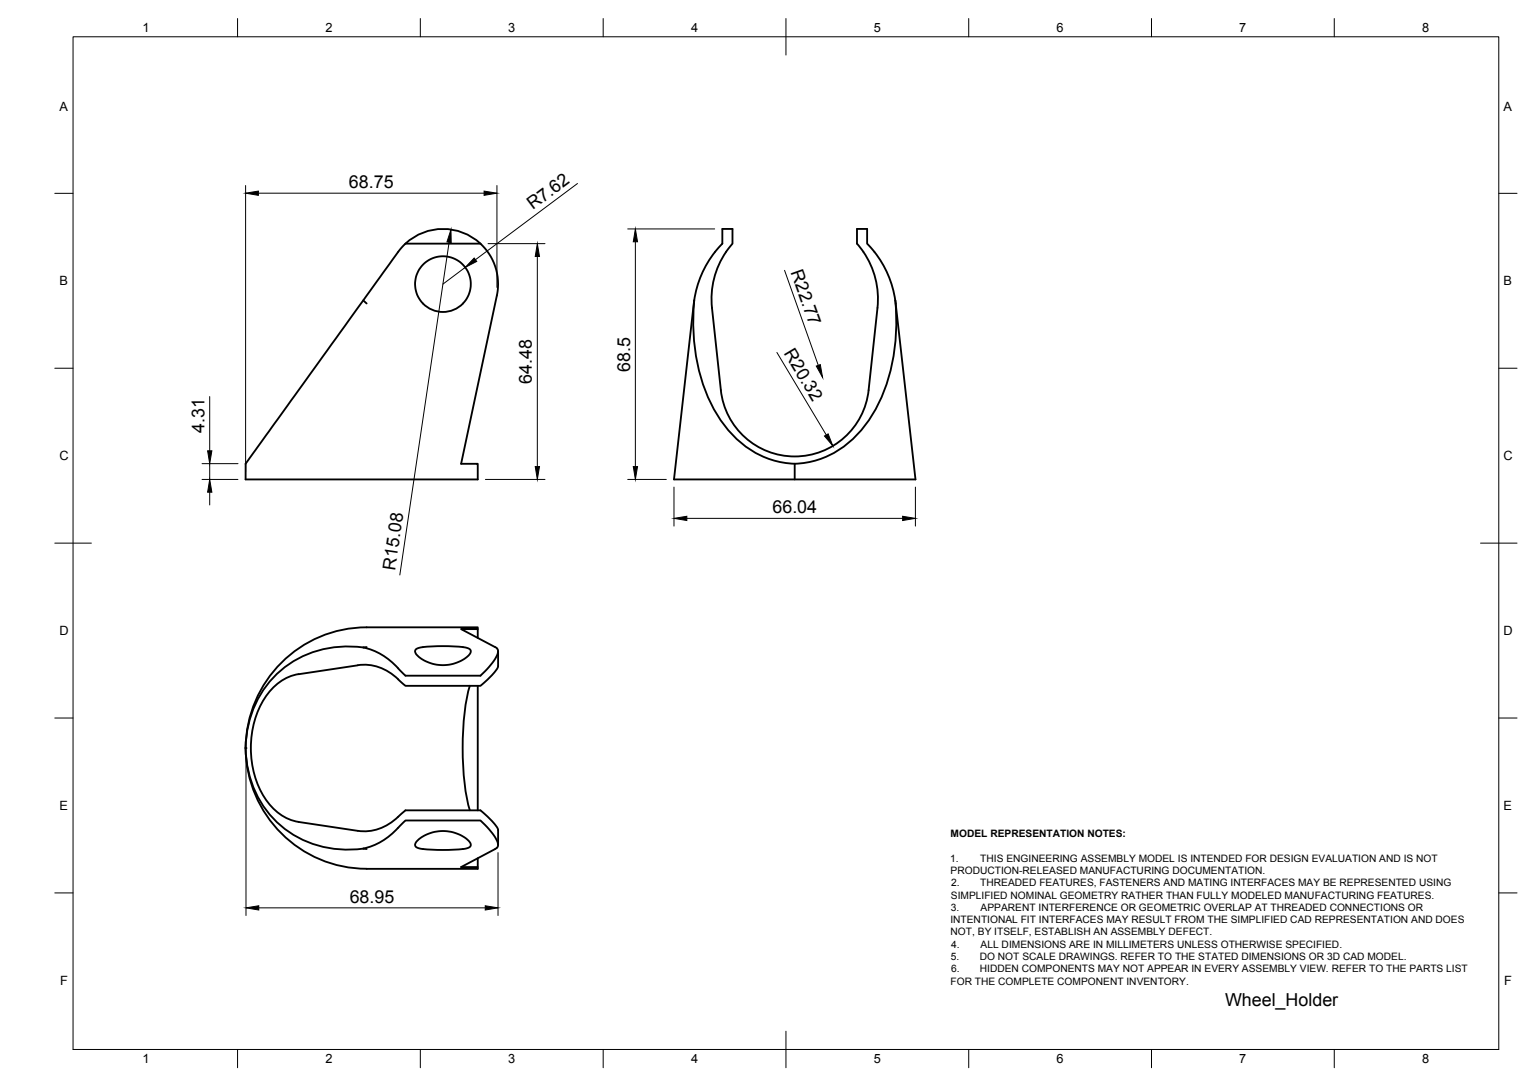
ISO-10303-21;
HEADER;
/* Generated by software containing ST-Developer
 * from STEP Tools, Inc. (www.steptools.com) 
 */

FILE_DESCRIPTION(
/* description */ ('Wheel Holder-Mirrored'),
/* implementation_level */ '2;1');

FILE_NAME(
/* name */ 'Wheel_Holder.step',
/* time_stamp */ '2026-10-07T09:01:46-07:00',
/* author */ (''),
/* organization */ (''),
/* preprocessor_version */ 'ST-DEVELOPER v20.2',
/* originating_system */ 'Autodesk Translation Framework v15.15.0.0',
/* authorisation */ '');

FILE_SCHEMA (('AUTOMOTIVE_DESIGN { 1 0 10303 214 3 1 1 }'));
ENDSEC;

DATA;
#10=MECHANICAL_DESIGN_GEOMETRIC_PRESENTATION_REPRESENTATION('',(#203),#3832);
#59=ELLIPSE('',#1988,0.00766814592499653,0.00762);
#60=ELLIPSE('',#1989,0.0076644002839305,0.00762);
#61=ELLIPSE('',#1993,0.0342294027026876,0.0277785949688766);
#62=ELLIPSE('',#1994,0.028399185304996,0.0277785949688766);
#63=ELLIPSE('',#2002,0.0232756976080203,0.0227670677706907);
#64=ELLIPSE('',#2003,0.0280540873991463,0.0227670677706907);
#65=ELLIPSE('',#2005,0.0232756976080203,0.0227670677706907);
#66=ELLIPSE('',#2006,0.0280540873991463,0.0227670677706907);
#67=ELLIPSE('',#2009,0.0207739608876574,0.02032);
#68=ELLIPSE('',#2010,0.0250387560529214,0.02032);
#69=ELLIPSE('',#2012,0.0076644002839305,0.00762);
#70=ELLIPSE('',#2016,0.0283991853049961,0.0277785949688767);
#71=ELLIPSE('',#2021,0.0570304735096183,0.0331133532215094);
#72=ELLIPSE('',#2022,0.0342294027026876,0.0277785949688767);
#73=ELLIPSE('',#2023,0.0570304735096183,0.0331133532215094);
#74=ELLIPSE('',#2025,0.0333225754026887,0.0331133532215094);
#75=ELLIPSE('',#2026,0.0333225754026887,0.0331133532215094);
#76=ELLIPSE('',#2028,0.00766814592499653,0.00762);
#77=ELLIPSE('',#2034,0.295962272640151,0.0331133532215094);
#170=B_SPLINE_CURVE_WITH_KNOTS('',3,(#3468,#3469,#3470,#3471,#3472,#3473,
#3474,#3475,#3476,#3477,#3478,#3479,#3480,#3481),.UNSPECIFIED.,.F.,.F.,
(4,2,2,2,2,2,4),(0.58453144748271,0.867768183831352,1.16094035782968,1.4691070433662,
1.77727372890272,2.07579244535874,2.37431116181475),.UNSPECIFIED.);
#171=B_SPLINE_CURVE_WITH_KNOTS('',3,(#3484,#3485,#3486,#3487,#3488,#3489,
#3490,#3491,#3492,#3493,#3494,#3495,#3496,#3497),.UNSPECIFIED.,.F.,.F.,
(4,2,2,2,2,2,4),(2.37431116181475,2.66483368462927,2.95535620744379,3.27144000918075,
3.58752381091772,3.88103472550587,4.16394043172282),.UNSPECIFIED.);
#172=B_SPLINE_CURVE_WITH_KNOTS('',3,(#3501,#3502,#3503,#3504,#3505,#3506,
#3507,#3508,#3509,#3510,#3511,#3512,#3513,#3514,#3515,#3516),
 .UNSPECIFIED.,.F.,.F.,(4,2,2,2,2,2,2,4),(-4.27790233879451,-4.09945168810992,
-3.81195458017329,-3.52445747223665,-3.22219845470822,-2.91993943717978,
-2.62905677671056,-2.33817411624134),.UNSPECIFIED.);
#173=B_SPLINE_CURVE_WITH_KNOTS('',3,(#3519,#3520,#3521,#3522,#3523,#3524,
#3525,#3526,#3527,#3528,#3529,#3530,#3531,#3532,#3533,#3534),
 .UNSPECIFIED.,.F.,.F.,(4,2,2,2,2,2,2,4),(-2.33817411624134,-2.04729145577211,
-1.75640879530289,-1.45414977777445,-1.15189076024602,-0.864393652309382,
-0.576896544372747,-0.398445893688138),.UNSPECIFIED.);
#174=B_SPLINE_CURVE_WITH_KNOTS('',3,(#3544,#3545,#3546,#3547,#3548,#3549,
#3550),.UNSPECIFIED.,.F.,.F.,(4,3,4),(-3.65201569549685,-3.58349548702897,
-3.30021421468191),.UNSPECIFIED.);
#175=B_SPLINE_CURVE_WITH_KNOTS('',3,(#3552,#3553,#3554,#3555,#3556,#3557,
#3558,#3559,#3560,#3561,#3562,#3563,#3564,#3565),.UNSPECIFIED.,.F.,.F.,
(4,2,2,2,2,2,4),(-7.77993041753592,-7.7480845912713,-7.46235224345222,-7.12519900195174,
-6.78804576045127,-6.11373927745031,-6.10347024465041),.UNSPECIFIED.);
#176=B_SPLINE_CURVE_WITH_KNOTS('',3,(#3596,#3597,#3598,#3599,#3600,#3601,
#3602,#3603,#3604,#3605,#3606,#3607,#3608,#3609),.UNSPECIFIED.,.F.,.F.,
(4,2,2,2,2,2,4),(-7.66118685225602,-7.63498959168202,-7.35041272704815,
-7.0310473742494,-6.71168202145065,-6.07295131585314,-6.03832591549393),
 .UNSPECIFIED.);
#177=B_SPLINE_CURVE_WITH_KNOTS('',3,(#3611,#3612,#3613,#3614,#3615,#3616),
 .UNSPECIFIED.,.F.,.F.,(4,2,4),(-3.62027438097633,-3.58564898061712,-3.28085403484185),
 .UNSPECIFIED.);
#178=B_SPLINE_CURVE_WITH_KNOTS('',3,(#3628,#3629,#3630,#3631,#3632,#3633,
#3634,#3635,#3636,#3637,#3638,#3639,#3640,#3641,#3642,#3643),
 .UNSPECIFIED.,.F.,.F.,(4,2,2,2,2,2,2,4),(0.398445893688145,0.576896544372747,
0.864393652309382,1.15189076024602,1.45414977777445,1.75640879530289,2.04729145577211,
2.33817411624133),.UNSPECIFIED.);
#179=B_SPLINE_CURVE_WITH_KNOTS('',3,(#3645,#3646,#3647,#3648,#3649,#3650,
#3651,#3652,#3653,#3654,#3655,#3656,#3657,#3658,#3659,#3660),
 .UNSPECIFIED.,.F.,.F.,(4,2,2,2,2,2,2,4),(2.33817411624133,2.62905677671056,
2.91993943717978,3.22219845470822,3.52445747223665,3.81195458017329,4.09945168810992,
4.27790233879452),.UNSPECIFIED.);
#180=B_SPLINE_CURVE_WITH_KNOTS('',3,(#3665,#3666,#3667,#3668,#3669,#3670),
 .UNSPECIFIED.,.F.,.F.,(4,2,4),(-6.38055499661601,-6.10670626645482,-6.04021537866389),
 .UNSPECIFIED.);
#181=B_SPLINE_CURVE_WITH_KNOTS('',3,(#3671,#3672,#3673,#3674,#3675,#3676,
#3677,#3678,#3679,#3680,#3681,#3682,#3683,#3684),.UNSPECIFIED.,.F.,.F.,
(4,2,2,2,2,2,4),(-3.62027438097633,-3.58564898061712,-2.94691827501961,
-2.62755292222086,-2.30818756942211,-2.02361070478824,-1.99741344421424),
 .UNSPECIFIED.);
#182=B_SPLINE_CURVE_WITH_KNOTS('',3,(#3724,#3725,#3726,#3727,#3728,#3729,
#3730),.UNSPECIFIED.,.F.,.F.,(4,3,4),(3.30021421468192,3.58349548702897,
3.65201569549685),.UNSPECIFIED.);
#183=B_SPLINE_CURVE_WITH_KNOTS('',3,(#3733,#3734,#3735,#3736,#3737,#3738,
#3739,#3740,#3741,#3742,#3743,#3744,#3745,#3746),.UNSPECIFIED.,.F.,.F.,
(4,2,2,2,2,2,4),(6.10060038618841,6.11086941898832,6.78517590198927,7.12232914348975,
7.45948238499022,7.7452147328093,7.77706055907392),.UNSPECIFIED.);
#184=B_SPLINE_CURVE_WITH_KNOTS('',3,(#3763,#3764,#3765,#3766,#3767,#3768,
#3769,#3770,#3771,#3772,#3773,#3774,#3775,#3776),.UNSPECIFIED.,.F.,.F.,
(4,2,2,2,2,2,4),(0.584524822753337,0.867430528970284,1.16094144355843,1.4770252452954,
1.79310904703237,2.08363156984688,2.3741540926614),.UNSPECIFIED.);
#185=B_SPLINE_CURVE_WITH_KNOTS('',3,(#3779,#3780,#3781,#3782,#3783,#3784,
#3785,#3786,#3787,#3788,#3789,#3790,#3791,#3792),.UNSPECIFIED.,.F.,.F.,
(4,2,2,2,2,2,4),(2.3741540926614,2.66467661547592,2.95519913829043,3.2712829400274,
3.58736674176437,3.88087765635252,4.16378336256947),.UNSPECIFIED.);
#191=SHAPE_REPRESENTATION_RELATIONSHIP('SRR','None',#3868,#197);
#197=ADVANCED_BREP_SHAPE_REPRESENTATION('',(#209),#3831);
#203=STYLED_ITEM('',(#3906),#209);
#209=MANIFOLD_SOLID_BREP('Body1',#1788);
#260=PLANE('',#1990);
#261=PLANE('',#1996);
#262=PLANE('',#1997);
#263=PLANE('',#1999);
#264=PLANE('',#2007);
#265=PLANE('',#2011);
#266=PLANE('',#2013);
#267=PLANE('',#2014);
#268=PLANE('',#2015);
#269=PLANE('',#2020);
#270=PLANE('',#2024);
#271=PLANE('',#2029);
#272=PLANE('',#2032);
#353=FACE_OUTER_BOUND('',#474,.T.);
#354=FACE_OUTER_BOUND('',#475,.T.);
#355=FACE_OUTER_BOUND('',#476,.T.);
#356=FACE_OUTER_BOUND('',#477,.T.);
#357=FACE_OUTER_BOUND('',#478,.T.);
#358=FACE_OUTER_BOUND('',#479,.T.);
#359=FACE_OUTER_BOUND('',#480,.T.);
#360=FACE_OUTER_BOUND('',#481,.T.);
#361=FACE_OUTER_BOUND('',#482,.T.);
#362=FACE_OUTER_BOUND('',#483,.T.);
#363=FACE_OUTER_BOUND('',#484,.T.);
#364=FACE_OUTER_BOUND('',#485,.T.);
#365=FACE_OUTER_BOUND('',#486,.T.);
#366=FACE_OUTER_BOUND('',#487,.T.);
#367=FACE_OUTER_BOUND('',#488,.T.);
#368=FACE_OUTER_BOUND('',#489,.T.);
#369=FACE_OUTER_BOUND('',#490,.T.);
#370=FACE_OUTER_BOUND('',#491,.T.);
#371=FACE_OUTER_BOUND('',#492,.T.);
#372=FACE_OUTER_BOUND('',#493,.T.);
#373=FACE_OUTER_BOUND('',#494,.T.);
#374=FACE_OUTER_BOUND('',#495,.T.);
#375=FACE_OUTER_BOUND('',#496,.T.);
#376=FACE_OUTER_BOUND('',#497,.T.);
#474=EDGE_LOOP('',(#1497,#1498,#1499,#1500,#1501,#1502,#1503,#1504));
#475=EDGE_LOOP('',(#1505,#1506));
#476=EDGE_LOOP('',(#1507,#1508,#1509,#1510,#1511,#1512,#1513,#1514,#1515,
#1516));
#477=EDGE_LOOP('',(#1517,#1518,#1519,#1520,#1521,#1522,#1523,#1524));
#478=EDGE_LOOP('',(#1525,#1526));
#479=EDGE_LOOP('',(#1527,#1528));
#480=EDGE_LOOP('',(#1529,#1530,#1531,#1532,#1533,#1534,#1535,#1536,#1537));
#481=EDGE_LOOP('',(#1538,#1539,#1540,#1541,#1542,#1543,#1544,#1545,#1546));
#482=EDGE_LOOP('',(#1547,#1548,#1549,#1550,#1551,#1552));
#483=EDGE_LOOP('',(#1553,#1554,#1555,#1556));
#484=EDGE_LOOP('',(#1557,#1558,#1559,#1560,#1561,#1562));
#485=EDGE_LOOP('',(#1563,#1564,#1565,#1566));
#486=EDGE_LOOP('',(#1567,#1568,#1569,#1570));
#487=EDGE_LOOP('',(#1571,#1572,#1573,#1574,#1575,#1576,#1577,#1578,#1579,
#1580,#1581,#1582));
#488=EDGE_LOOP('',(#1583,#1584,#1585,#1586,#1587,#1588,#1589,#1590));
#489=EDGE_LOOP('',(#1591,#1592,#1593,#1594,#1595,#1596,#1597,#1598));
#490=EDGE_LOOP('',(#1599,#1600,#1601,#1602,#1603,#1604,#1605,#1606,#1607,
#1608,#1609));
#491=EDGE_LOOP('',(#1610,#1611,#1612,#1613,#1614));
#492=EDGE_LOOP('',(#1615,#1616,#1617,#1618,#1619,#1620,#1621,#1622));
#493=EDGE_LOOP('',(#1623,#1624));
#494=EDGE_LOOP('',(#1625,#1626,#1627,#1628,#1629,#1630,#1631,#1632,#1633,
#1634));
#495=EDGE_LOOP('',(#1635,#1636,#1637,#1638,#1639,#1640,#1641,#1642));
#496=EDGE_LOOP('',(#1643,#1644,#1645,#1646,#1647));
#497=EDGE_LOOP('',(#1648,#1649,#1650,#1651,#1652));
#554=LINE('',#3499,#647);
#555=LINE('',#3538,#648);
#556=LINE('',#3568,#649);
#557=LINE('',#3570,#650);
#558=LINE('',#3574,#651);
#559=LINE('',#3576,#652);
#560=LINE('',#3578,#653);
#561=LINE('',#3580,#654);
#562=LINE('',#3581,#655);
#563=LINE('',#3585,#656);
#564=LINE('',#3591,#657);
#565=LINE('',#3619,#658);
#566=LINE('',#3620,#659);
#567=LINE('',#3626,#660);
#568=LINE('',#3662,#661);
#569=LINE('',#3688,#662);
#570=LINE('',#3689,#663);
#571=LINE('',#3690,#664);
#572=LINE('',#3696,#665);
#573=LINE('',#3698,#666);
#574=LINE('',#3699,#667);
#575=LINE('',#3703,#668);
#576=LINE('',#3705,#669);
#577=LINE('',#3706,#670);
#578=LINE('',#3709,#671);
#579=LINE('',#3710,#672);
#580=LINE('',#3713,#673);
#581=LINE('',#3716,#674);
#582=LINE('',#3717,#675);
#583=LINE('',#3719,#676);
#584=LINE('',#3722,#677);
#585=LINE('',#3755,#678);
#586=LINE('',#3761,#679);
#587=LINE('',#3794,#680);
#588=LINE('',#3797,#681);
#589=LINE('',#3798,#682);
#590=LINE('',#3801,#683);
#647=VECTOR('',#2370,0.00762);
#648=VECTOR('',#2375,1.);
#649=VECTOR('',#2384,1.);
#650=VECTOR('',#2385,1.);
#651=VECTOR('',#2390,1.);
#652=VECTOR('',#2391,1.);
#653=VECTOR('',#2392,1.);
#654=VECTOR('',#2393,1.);
#655=VECTOR('',#2394,1.);
#656=VECTOR('',#2397,1.);
#657=VECTOR('',#2404,1.);
#658=VECTOR('',#2411,1.);
#659=VECTOR('',#2412,1.);
#660=VECTOR('',#2417,1.);
#661=VECTOR('',#2418,1.);
#662=VECTOR('',#2423,1.);
#663=VECTOR('',#2424,1.);
#664=VECTOR('',#2425,1.);
#665=VECTOR('',#2432,1.);
#666=VECTOR('',#2435,1.);
#667=VECTOR('',#2436,1.);
#668=VECTOR('',#2441,1.);
#669=VECTOR('',#2442,1.);
#670=VECTOR('',#2443,1.);
#671=VECTOR('',#2446,1.);
#672=VECTOR('',#2447,1.);
#673=VECTOR('',#2450,1.);
#674=VECTOR('',#2453,1.);
#675=VECTOR('',#2454,1.);
#676=VECTOR('',#2457,1.);
#677=VECTOR('',#2460,1.);
#678=VECTOR('',#2473,1.);
#679=VECTOR('',#2480,0.00762);
#680=VECTOR('',#2485,1.);
#681=VECTOR('',#2488,1.);
#682=VECTOR('',#2489,1.);
#683=VECTOR('',#2494,1.);
#740=CIRCLE('',#1991,0.01508125);
#741=CIRCLE('',#1995,0.0608802828924915);
#742=CIRCLE('',#1998,0.01508125);
#743=CIRCLE('',#2000,0.01508125);
#744=CIRCLE('',#2019,0.01508125);
#745=CIRCLE('',#2031,0.0608802828794672);
#851=VERTEX_POINT('',#3466);
#852=VERTEX_POINT('',#3467);
#853=VERTEX_POINT('',#3482);
#854=VERTEX_POINT('',#3498);
#855=VERTEX_POINT('',#3500);
#856=VERTEX_POINT('',#3517);
#857=VERTEX_POINT('',#3536);
#858=VERTEX_POINT('',#3537);
#859=VERTEX_POINT('',#3541);
#860=VERTEX_POINT('',#3542);
#861=VERTEX_POINT('',#3551);
#862=VERTEX_POINT('',#3566);
#863=VERTEX_POINT('',#3569);
#864=VERTEX_POINT('',#3573);
#865=VERTEX_POINT('',#3575);
#866=VERTEX_POINT('',#3577);
#867=VERTEX_POINT('',#3579);
#868=VERTEX_POINT('',#3583);
#869=VERTEX_POINT('',#3584);
#870=VERTEX_POINT('',#3588);
#871=VERTEX_POINT('',#3589);
#872=VERTEX_POINT('',#3593);
#873=VERTEX_POINT('',#3594);
#874=VERTEX_POINT('',#3610);
#875=VERTEX_POINT('',#3617);
#876=VERTEX_POINT('',#3622);
#877=VERTEX_POINT('',#3623);
#878=VERTEX_POINT('',#3625);
#879=VERTEX_POINT('',#3627);
#880=VERTEX_POINT('',#3644);
#881=VERTEX_POINT('',#3661);
#882=VERTEX_POINT('',#3663);
#883=VERTEX_POINT('',#3686);
#884=VERTEX_POINT('',#3687);
#885=VERTEX_POINT('',#3692);
#886=VERTEX_POINT('',#3694);
#887=VERTEX_POINT('',#3702);
#888=VERTEX_POINT('',#3704);
#889=VERTEX_POINT('',#3708);
#890=VERTEX_POINT('',#3712);
#891=VERTEX_POINT('',#3714);
#892=VERTEX_POINT('',#3721);
#893=VERTEX_POINT('',#3723);
#894=VERTEX_POINT('',#3731);
#895=VERTEX_POINT('',#3748);
#896=VERTEX_POINT('',#3749);
#897=VERTEX_POINT('',#3754);
#898=VERTEX_POINT('',#3756);
#899=VERTEX_POINT('',#3760);
#900=VERTEX_POINT('',#3762);
#901=VERTEX_POINT('',#3777);
#902=VERTEX_POINT('',#3796);
#1075=EDGE_CURVE('',#851,#852,#170,.T.);
#1076=EDGE_CURVE('',#853,#851,#59,.T.);
#1077=EDGE_CURVE('',#852,#853,#171,.T.);
#1078=EDGE_CURVE('',#852,#854,#554,.T.);
#1079=EDGE_CURVE('',#854,#855,#172,.F.);
#1080=EDGE_CURVE('',#856,#855,#60,.T.);
#1081=EDGE_CURVE('',#856,#854,#173,.F.);
#1082=EDGE_CURVE('',#857,#858,#555,.T.);
#1083=EDGE_CURVE('',#857,#858,#740,.T.);
#1084=EDGE_CURVE('',#859,#860,#61,.T.);
#1085=EDGE_CURVE('',#857,#860,#174,.T.);
#1086=EDGE_CURVE('',#861,#858,#175,.T.);
#1087=EDGE_CURVE('',#861,#862,#62,.T.);
#1088=EDGE_CURVE('',#851,#862,#556,.T.);
#1089=EDGE_CURVE('',#863,#853,#557,.T.);
#1090=EDGE_CURVE('',#859,#863,#741,.T.);
#1091=EDGE_CURVE('',#862,#864,#558,.T.);
#1092=EDGE_CURVE('',#864,#865,#559,.T.);
#1093=EDGE_CURVE('',#865,#866,#560,.T.);
#1094=EDGE_CURVE('',#867,#866,#561,.T.);
#1095=EDGE_CURVE('',#863,#867,#562,.F.);
#1096=EDGE_CURVE('',#868,#869,#563,.T.);
#1097=EDGE_CURVE('',#868,#869,#742,.T.);
#1098=EDGE_CURVE('',#870,#871,#743,.T.);
#1099=EDGE_CURVE('',#871,#870,#564,.T.);
#1100=EDGE_CURVE('',#872,#873,#63,.T.);
#1101=EDGE_CURVE('',#872,#870,#176,.T.);
#1102=EDGE_CURVE('',#871,#874,#177,.T.);
#1103=EDGE_CURVE('',#875,#874,#64,.T.);
#1104=EDGE_CURVE('',#875,#855,#565,.T.);
#1105=EDGE_CURVE('',#856,#873,#566,.T.);
#1106=EDGE_CURVE('',#876,#877,#65,.T.);
#1107=EDGE_CURVE('',#878,#876,#567,.T.);
#1108=EDGE_CURVE('',#879,#878,#178,.F.);
#1109=EDGE_CURVE('',#880,#879,#179,.F.);
#1110=EDGE_CURVE('',#881,#880,#568,.T.);
#1111=EDGE_CURVE('',#882,#881,#66,.T.);
#1112=EDGE_CURVE('',#882,#868,#180,.T.);
#1113=EDGE_CURVE('',#869,#877,#181,.T.);
#1114=EDGE_CURVE('',#883,#884,#569,.T.);
#1115=EDGE_CURVE('',#884,#873,#570,.T.);
#1116=EDGE_CURVE('',#875,#883,#571,.T.);
#1117=EDGE_CURVE('',#884,#885,#67,.T.);
#1118=EDGE_CURVE('',#886,#883,#68,.T.);
#1119=EDGE_CURVE('',#886,#885,#572,.T.);
#1120=EDGE_CURVE('',#885,#876,#573,.T.);
#1121=EDGE_CURVE('',#881,#886,#574,.T.);
#1122=EDGE_CURVE('',#878,#880,#69,.T.);
#1123=EDGE_CURVE('',#865,#887,#575,.T.);
#1124=EDGE_CURVE('',#888,#887,#576,.T.);
#1125=EDGE_CURVE('',#866,#888,#577,.T.);
#1126=EDGE_CURVE('',#864,#889,#578,.T.);
#1127=EDGE_CURVE('',#887,#889,#579,.T.);
#1128=EDGE_CURVE('',#877,#890,#580,.T.);
#1129=EDGE_CURVE('',#891,#890,#70,.T.);
#1130=EDGE_CURVE('',#889,#891,#581,.T.);
#1131=EDGE_CURVE('',#861,#872,#582,.T.);
#1132=EDGE_CURVE('',#860,#874,#583,.T.);
#1133=EDGE_CURVE('',#882,#892,#584,.T.);
#1134=EDGE_CURVE('',#892,#893,#182,.T.);
#1135=EDGE_CURVE('',#894,#893,#744,.T.);
#1136=EDGE_CURVE('',#894,#890,#183,.T.);
#1137=EDGE_CURVE('',#895,#896,#71,.T.);
#1138=EDGE_CURVE('',#892,#895,#72,.T.);
#1139=EDGE_CURVE('',#896,#859,#73,.T.);
#1140=EDGE_CURVE('',#897,#888,#585,.T.);
#1141=EDGE_CURVE('',#898,#897,#74,.F.);
#1142=EDGE_CURVE('',#867,#898,#75,.F.);
#1143=EDGE_CURVE('',#879,#899,#586,.T.);
#1144=EDGE_CURVE('',#900,#899,#184,.T.);
#1145=EDGE_CURVE('',#901,#900,#76,.T.);
#1146=EDGE_CURVE('',#899,#901,#185,.T.);
#1147=EDGE_CURVE('',#893,#894,#587,.T.);
#1148=EDGE_CURVE('',#902,#900,#588,.T.);
#1149=EDGE_CURVE('',#901,#891,#589,.T.);
#1150=EDGE_CURVE('',#902,#895,#745,.F.);
#1151=EDGE_CURVE('',#897,#902,#590,.F.);
#1152=EDGE_CURVE('',#896,#898,#77,.F.);
#1497=ORIENTED_EDGE('',*,*,#1075,.F.);
#1498=ORIENTED_EDGE('',*,*,#1076,.F.);
#1499=ORIENTED_EDGE('',*,*,#1077,.F.);
#1500=ORIENTED_EDGE('',*,*,#1078,.T.);
#1501=ORIENTED_EDGE('',*,*,#1079,.T.);
#1502=ORIENTED_EDGE('',*,*,#1080,.F.);
#1503=ORIENTED_EDGE('',*,*,#1081,.T.);
#1504=ORIENTED_EDGE('',*,*,#1078,.F.);
#1505=ORIENTED_EDGE('',*,*,#1082,.F.);
#1506=ORIENTED_EDGE('',*,*,#1083,.T.);
#1507=ORIENTED_EDGE('',*,*,#1084,.T.);
#1508=ORIENTED_EDGE('',*,*,#1085,.F.);
#1509=ORIENTED_EDGE('',*,*,#1082,.T.);
#1510=ORIENTED_EDGE('',*,*,#1086,.F.);
#1511=ORIENTED_EDGE('',*,*,#1087,.T.);
#1512=ORIENTED_EDGE('',*,*,#1088,.F.);
#1513=ORIENTED_EDGE('',*,*,#1075,.T.);
#1514=ORIENTED_EDGE('',*,*,#1077,.T.);
#1515=ORIENTED_EDGE('',*,*,#1089,.F.);
#1516=ORIENTED_EDGE('',*,*,#1090,.F.);
#1517=ORIENTED_EDGE('',*,*,#1089,.T.);
#1518=ORIENTED_EDGE('',*,*,#1076,.T.);
#1519=ORIENTED_EDGE('',*,*,#1088,.T.);
#1520=ORIENTED_EDGE('',*,*,#1091,.T.);
#1521=ORIENTED_EDGE('',*,*,#1092,.T.);
#1522=ORIENTED_EDGE('',*,*,#1093,.T.);
#1523=ORIENTED_EDGE('',*,*,#1094,.F.);
#1524=ORIENTED_EDGE('',*,*,#1095,.F.);
#1525=ORIENTED_EDGE('',*,*,#1096,.F.);
#1526=ORIENTED_EDGE('',*,*,#1097,.T.);
#1527=ORIENTED_EDGE('',*,*,#1098,.T.);
#1528=ORIENTED_EDGE('',*,*,#1099,.T.);
#1529=ORIENTED_EDGE('',*,*,#1100,.F.);
#1530=ORIENTED_EDGE('',*,*,#1101,.T.);
#1531=ORIENTED_EDGE('',*,*,#1099,.F.);
#1532=ORIENTED_EDGE('',*,*,#1102,.T.);
#1533=ORIENTED_EDGE('',*,*,#1103,.F.);
#1534=ORIENTED_EDGE('',*,*,#1104,.T.);
#1535=ORIENTED_EDGE('',*,*,#1079,.F.);
#1536=ORIENTED_EDGE('',*,*,#1081,.F.);
#1537=ORIENTED_EDGE('',*,*,#1105,.T.);
#1538=ORIENTED_EDGE('',*,*,#1106,.F.);
#1539=ORIENTED_EDGE('',*,*,#1107,.F.);
#1540=ORIENTED_EDGE('',*,*,#1108,.F.);
#1541=ORIENTED_EDGE('',*,*,#1109,.F.);
#1542=ORIENTED_EDGE('',*,*,#1110,.F.);
#1543=ORIENTED_EDGE('',*,*,#1111,.F.);
#1544=ORIENTED_EDGE('',*,*,#1112,.T.);
#1545=ORIENTED_EDGE('',*,*,#1096,.T.);
#1546=ORIENTED_EDGE('',*,*,#1113,.T.);
#1547=ORIENTED_EDGE('',*,*,#1114,.T.);
#1548=ORIENTED_EDGE('',*,*,#1115,.T.);
#1549=ORIENTED_EDGE('',*,*,#1105,.F.);
#1550=ORIENTED_EDGE('',*,*,#1080,.T.);
#1551=ORIENTED_EDGE('',*,*,#1104,.F.);
#1552=ORIENTED_EDGE('',*,*,#1116,.T.);
#1553=ORIENTED_EDGE('',*,*,#1117,.F.);
#1554=ORIENTED_EDGE('',*,*,#1114,.F.);
#1555=ORIENTED_EDGE('',*,*,#1118,.F.);
#1556=ORIENTED_EDGE('',*,*,#1119,.T.);
#1557=ORIENTED_EDGE('',*,*,#1120,.F.);
#1558=ORIENTED_EDGE('',*,*,#1119,.F.);
#1559=ORIENTED_EDGE('',*,*,#1121,.F.);
#1560=ORIENTED_EDGE('',*,*,#1110,.T.);
#1561=ORIENTED_EDGE('',*,*,#1122,.F.);
#1562=ORIENTED_EDGE('',*,*,#1107,.T.);
#1563=ORIENTED_EDGE('',*,*,#1123,.T.);
#1564=ORIENTED_EDGE('',*,*,#1124,.F.);
#1565=ORIENTED_EDGE('',*,*,#1125,.F.);
#1566=ORIENTED_EDGE('',*,*,#1093,.F.);
#1567=ORIENTED_EDGE('',*,*,#1126,.T.);
#1568=ORIENTED_EDGE('',*,*,#1127,.F.);
#1569=ORIENTED_EDGE('',*,*,#1123,.F.);
#1570=ORIENTED_EDGE('',*,*,#1092,.F.);
#1571=ORIENTED_EDGE('',*,*,#1100,.T.);
#1572=ORIENTED_EDGE('',*,*,#1115,.F.);
#1573=ORIENTED_EDGE('',*,*,#1117,.T.);
#1574=ORIENTED_EDGE('',*,*,#1120,.T.);
#1575=ORIENTED_EDGE('',*,*,#1106,.T.);
#1576=ORIENTED_EDGE('',*,*,#1128,.T.);
#1577=ORIENTED_EDGE('',*,*,#1129,.F.);
#1578=ORIENTED_EDGE('',*,*,#1130,.F.);
#1579=ORIENTED_EDGE('',*,*,#1126,.F.);
#1580=ORIENTED_EDGE('',*,*,#1091,.F.);
#1581=ORIENTED_EDGE('',*,*,#1087,.F.);
#1582=ORIENTED_EDGE('',*,*,#1131,.T.);
#1583=ORIENTED_EDGE('',*,*,#1101,.F.);
#1584=ORIENTED_EDGE('',*,*,#1131,.F.);
#1585=ORIENTED_EDGE('',*,*,#1086,.T.);
#1586=ORIENTED_EDGE('',*,*,#1083,.F.);
#1587=ORIENTED_EDGE('',*,*,#1085,.T.);
#1588=ORIENTED_EDGE('',*,*,#1132,.T.);
#1589=ORIENTED_EDGE('',*,*,#1102,.F.);
#1590=ORIENTED_EDGE('',*,*,#1098,.F.);
#1591=ORIENTED_EDGE('',*,*,#1133,.T.);
#1592=ORIENTED_EDGE('',*,*,#1134,.T.);
#1593=ORIENTED_EDGE('',*,*,#1135,.F.);
#1594=ORIENTED_EDGE('',*,*,#1136,.T.);
#1595=ORIENTED_EDGE('',*,*,#1128,.F.);
#1596=ORIENTED_EDGE('',*,*,#1113,.F.);
#1597=ORIENTED_EDGE('',*,*,#1097,.F.);
#1598=ORIENTED_EDGE('',*,*,#1112,.F.);
#1599=ORIENTED_EDGE('',*,*,#1137,.F.);
#1600=ORIENTED_EDGE('',*,*,#1138,.F.);
#1601=ORIENTED_EDGE('',*,*,#1133,.F.);
#1602=ORIENTED_EDGE('',*,*,#1111,.T.);
#1603=ORIENTED_EDGE('',*,*,#1121,.T.);
#1604=ORIENTED_EDGE('',*,*,#1118,.T.);
#1605=ORIENTED_EDGE('',*,*,#1116,.F.);
#1606=ORIENTED_EDGE('',*,*,#1103,.T.);
#1607=ORIENTED_EDGE('',*,*,#1132,.F.);
#1608=ORIENTED_EDGE('',*,*,#1084,.F.);
#1609=ORIENTED_EDGE('',*,*,#1139,.F.);
#1610=ORIENTED_EDGE('',*,*,#1094,.T.);
#1611=ORIENTED_EDGE('',*,*,#1125,.T.);
#1612=ORIENTED_EDGE('',*,*,#1140,.F.);
#1613=ORIENTED_EDGE('',*,*,#1141,.F.);
#1614=ORIENTED_EDGE('',*,*,#1142,.F.);
#1615=ORIENTED_EDGE('',*,*,#1109,.T.);
#1616=ORIENTED_EDGE('',*,*,#1143,.T.);
#1617=ORIENTED_EDGE('',*,*,#1144,.F.);
#1618=ORIENTED_EDGE('',*,*,#1145,.F.);
#1619=ORIENTED_EDGE('',*,*,#1146,.F.);
#1620=ORIENTED_EDGE('',*,*,#1143,.F.);
#1621=ORIENTED_EDGE('',*,*,#1108,.T.);
#1622=ORIENTED_EDGE('',*,*,#1122,.T.);
#1623=ORIENTED_EDGE('',*,*,#1135,.T.);
#1624=ORIENTED_EDGE('',*,*,#1147,.T.);
#1625=ORIENTED_EDGE('',*,*,#1148,.T.);
#1626=ORIENTED_EDGE('',*,*,#1144,.T.);
#1627=ORIENTED_EDGE('',*,*,#1146,.T.);
#1628=ORIENTED_EDGE('',*,*,#1149,.T.);
#1629=ORIENTED_EDGE('',*,*,#1129,.T.);
#1630=ORIENTED_EDGE('',*,*,#1136,.F.);
#1631=ORIENTED_EDGE('',*,*,#1147,.F.);
#1632=ORIENTED_EDGE('',*,*,#1134,.F.);
#1633=ORIENTED_EDGE('',*,*,#1138,.T.);
#1634=ORIENTED_EDGE('',*,*,#1150,.F.);
#1635=ORIENTED_EDGE('',*,*,#1140,.T.);
#1636=ORIENTED_EDGE('',*,*,#1124,.T.);
#1637=ORIENTED_EDGE('',*,*,#1127,.T.);
#1638=ORIENTED_EDGE('',*,*,#1130,.T.);
#1639=ORIENTED_EDGE('',*,*,#1149,.F.);
#1640=ORIENTED_EDGE('',*,*,#1145,.T.);
#1641=ORIENTED_EDGE('',*,*,#1148,.F.);
#1642=ORIENTED_EDGE('',*,*,#1151,.F.);
#1643=ORIENTED_EDGE('',*,*,#1151,.T.);
#1644=ORIENTED_EDGE('',*,*,#1150,.T.);
#1645=ORIENTED_EDGE('',*,*,#1137,.T.);
#1646=ORIENTED_EDGE('',*,*,#1152,.T.);
#1647=ORIENTED_EDGE('',*,*,#1141,.T.);
#1648=ORIENTED_EDGE('',*,*,#1142,.T.);
#1649=ORIENTED_EDGE('',*,*,#1152,.F.);
#1650=ORIENTED_EDGE('',*,*,#1139,.T.);
#1651=ORIENTED_EDGE('',*,*,#1090,.T.);
#1652=ORIENTED_EDGE('',*,*,#1095,.T.);
#1668=CYLINDRICAL_SURFACE('',#1987,0.00762);
#1669=CYLINDRICAL_SURFACE('',#1992,0.0277785949688766);
#1670=CYLINDRICAL_SURFACE('',#2001,0.0227670677706907);
#1671=CYLINDRICAL_SURFACE('',#2004,0.0227670677706907);
#1672=CYLINDRICAL_SURFACE('',#2008,0.02032);
#1673=CYLINDRICAL_SURFACE('',#2017,0.01508125);
#1674=CYLINDRICAL_SURFACE('',#2018,0.01508125);
#1675=CYLINDRICAL_SURFACE('',#2027,0.00762);
#1676=CYLINDRICAL_SURFACE('',#2030,0.0277785949688767);
#1677=CYLINDRICAL_SURFACE('',#2033,0.0331133532215094);
#1678=CYLINDRICAL_SURFACE('',#2035,0.0331133532215094);
#1759=ADVANCED_FACE('',(#353),#1668,.F.);
#1760=ADVANCED_FACE('',(#354),#260,.F.);
#1761=ADVANCED_FACE('',(#355),#1669,.T.);
#1762=ADVANCED_FACE('',(#356),#261,.T.);
#1763=ADVANCED_FACE('',(#357),#262,.F.);
#1764=ADVANCED_FACE('',(#358),#263,.F.);
#1765=ADVANCED_FACE('',(#359),#1670,.F.);
#1766=ADVANCED_FACE('',(#360),#1671,.F.);
#1767=ADVANCED_FACE('',(#361),#264,.T.);
#1768=ADVANCED_FACE('',(#362),#1672,.F.);
#1769=ADVANCED_FACE('',(#363),#265,.F.);
#1770=ADVANCED_FACE('',(#364),#266,.T.);
#1771=ADVANCED_FACE('',(#365),#267,.T.);
#1772=ADVANCED_FACE('',(#366),#268,.T.);
#1773=ADVANCED_FACE('',(#367),#1673,.T.);
#1774=ADVANCED_FACE('',(#368),#1674,.T.);
#1775=ADVANCED_FACE('',(#369),#269,.T.);
#1776=ADVANCED_FACE('',(#370),#270,.F.);
#1777=ADVANCED_FACE('',(#371),#1675,.F.);
#1778=ADVANCED_FACE('',(#372),#271,.F.);
#1779=ADVANCED_FACE('',(#373),#1676,.T.);
#1780=ADVANCED_FACE('',(#374),#272,.T.);
#1781=ADVANCED_FACE('',(#375),#1677,.T.);
#1782=ADVANCED_FACE('',(#376),#1678,.T.);
#1788=CLOSED_SHELL('',(#1759,#1760,#1761,#1762,#1763,#1764,#1765,#1766,
#1767,#1768,#1769,#1770,#1771,#1772,#1773,#1774,#1775,#1776,#1777,#1778,
#1779,#1780,#1781,#1782));
#1986=AXIS2_PLACEMENT_3D('',#3464,#2364,#2365);
#1987=AXIS2_PLACEMENT_3D('',#3465,#2366,#2367);
#1988=AXIS2_PLACEMENT_3D('',#3483,#2368,#2369);
#1989=AXIS2_PLACEMENT_3D('',#3518,#2371,#2372);
#1990=AXIS2_PLACEMENT_3D('',#3535,#2373,#2374);
#1991=AXIS2_PLACEMENT_3D('',#3539,#2376,#2377);
#1992=AXIS2_PLACEMENT_3D('',#3540,#2378,#2379);
#1993=AXIS2_PLACEMENT_3D('',#3543,#2380,#2381);
#1994=AXIS2_PLACEMENT_3D('',#3567,#2382,#2383);
#1995=AXIS2_PLACEMENT_3D('',#3571,#2386,#2387);
#1996=AXIS2_PLACEMENT_3D('',#3572,#2388,#2389);
#1997=AXIS2_PLACEMENT_3D('',#3582,#2395,#2396);
#1998=AXIS2_PLACEMENT_3D('',#3586,#2398,#2399);
#1999=AXIS2_PLACEMENT_3D('',#3587,#2400,#2401);
#2000=AXIS2_PLACEMENT_3D('',#3590,#2402,#2403);
#2001=AXIS2_PLACEMENT_3D('',#3592,#2405,#2406);
#2002=AXIS2_PLACEMENT_3D('',#3595,#2407,#2408);
#2003=AXIS2_PLACEMENT_3D('',#3618,#2409,#2410);
#2004=AXIS2_PLACEMENT_3D('',#3621,#2413,#2414);
#2005=AXIS2_PLACEMENT_3D('',#3624,#2415,#2416);
#2006=AXIS2_PLACEMENT_3D('',#3664,#2419,#2420);
#2007=AXIS2_PLACEMENT_3D('',#3685,#2421,#2422);
#2008=AXIS2_PLACEMENT_3D('',#3691,#2426,#2427);
#2009=AXIS2_PLACEMENT_3D('',#3693,#2428,#2429);
#2010=AXIS2_PLACEMENT_3D('',#3695,#2430,#2431);
#2011=AXIS2_PLACEMENT_3D('',#3697,#2433,#2434);
#2012=AXIS2_PLACEMENT_3D('',#3700,#2437,#2438);
#2013=AXIS2_PLACEMENT_3D('',#3701,#2439,#2440);
#2014=AXIS2_PLACEMENT_3D('',#3707,#2444,#2445);
#2015=AXIS2_PLACEMENT_3D('',#3711,#2448,#2449);
#2016=AXIS2_PLACEMENT_3D('',#3715,#2451,#2452);
#2017=AXIS2_PLACEMENT_3D('',#3718,#2455,#2456);
#2018=AXIS2_PLACEMENT_3D('',#3720,#2458,#2459);
#2019=AXIS2_PLACEMENT_3D('',#3732,#2461,#2462);
#2020=AXIS2_PLACEMENT_3D('',#3747,#2463,#2464);
#2021=AXIS2_PLACEMENT_3D('',#3750,#2465,#2466);
#2022=AXIS2_PLACEMENT_3D('',#3751,#2467,#2468);
#2023=AXIS2_PLACEMENT_3D('',#3752,#2469,#2470);
#2024=AXIS2_PLACEMENT_3D('',#3753,#2471,#2472);
#2025=AXIS2_PLACEMENT_3D('',#3757,#2474,#2475);
#2026=AXIS2_PLACEMENT_3D('',#3758,#2476,#2477);
#2027=AXIS2_PLACEMENT_3D('',#3759,#2478,#2479);
#2028=AXIS2_PLACEMENT_3D('',#3778,#2481,#2482);
#2029=AXIS2_PLACEMENT_3D('',#3793,#2483,#2484);
#2030=AXIS2_PLACEMENT_3D('',#3795,#2486,#2487);
#2031=AXIS2_PLACEMENT_3D('',#3799,#2490,#2491);
#2032=AXIS2_PLACEMENT_3D('',#3800,#2492,#2493);
#2033=AXIS2_PLACEMENT_3D('',#3802,#2495,#2496);
#2034=AXIS2_PLACEMENT_3D('',#3803,#2497,#2498);
#2035=AXIS2_PLACEMENT_3D('',#3804,#2499,#2500);
#2364=DIRECTION('axis',(0.,0.,1.));
#2365=DIRECTION('refdir',(1.,0.,0.));
#2366=DIRECTION('center_axis',(-1.,0.,0.));
#2367=DIRECTION('ref_axis',(0.,0.,-1.));
#2368=DIRECTION('center_axis',(-0.99372130819269,0.,-0.111883696952722));
#2369=DIRECTION('ref_axis',(-0.111883696952722,0.,0.99372130819269));
#2370=DIRECTION('',(-1.,0.,0.));
#2371=DIRECTION('center_axis',(0.994206946103325,0.,-0.107482781504297));
#2372=DIRECTION('ref_axis',(-0.107482781504297,0.,-0.994206946103325));
#2373=DIRECTION('center_axis',(-1.,0.,0.));
#2374=DIRECTION('ref_axis',(0.,0.,-1.));
#2375=DIRECTION('',(0.,-1.,0.));
#2376=DIRECTION('center_axis',(1.,0.,0.));
#2377=DIRECTION('ref_axis',(0.,0.,-1.));
#2378=DIRECTION('center_axis',(0.,-1.,0.));
#2379=DIRECTION('ref_axis',(0.,0.,1.));
#2380=DIRECTION('center_axis',(0.,-0.811541913546029,-0.5842942089034));
#2381=DIRECTION('ref_axis',(0.,-0.5842942089034,0.811541913546029));
#2382=DIRECTION('center_axis',(0.,0.978147600733806,0.207911690817759));
#2383=DIRECTION('ref_axis',(0.,-0.207911690817759,0.978147600733806));
#2384=DIRECTION('',(0.,-1.,0.));
#2385=DIRECTION('',(0.,-1.,0.));
#2386=DIRECTION('center_axis',(0.0838731411310077,0.675424884631005,-0.732643515918903));
#2387=DIRECTION('ref_axis',(0.993606931693314,-0.000929786476276916,0.112891101456694));
#2388=DIRECTION('center_axis',(0.99372130819269,0.,0.111883696952722));
#2389=DIRECTION('ref_axis',(-0.111883696952722,0.,0.99372130819269));
#2390=DIRECTION('',(0.109468391364691,0.206662199202023,-0.97226920485687));
#2391=DIRECTION('',(0.,-1.,0.));
#2392=DIRECTION('',(0.111883696952722,0.,-0.99372130819269));
#2393=DIRECTION('',(0.,-1.,0.));
#2394=DIRECTION('',(-0.111883696952722,0.,0.99372130819269));
#2395=DIRECTION('center_axis',(-1.,0.,0.));
#2396=DIRECTION('ref_axis',(0.,0.,-1.));
#2397=DIRECTION('',(0.,-1.,0.));
#2398=DIRECTION('center_axis',(1.,0.,0.));
#2399=DIRECTION('ref_axis',(0.,0.,-1.));
#2400=DIRECTION('center_axis',(1.,0.,0.));
#2401=DIRECTION('ref_axis',(0.,0.,1.));
#2402=DIRECTION('center_axis',(-1.,0.,0.));
#2403=DIRECTION('ref_axis',(0.,0.,1.));
#2404=DIRECTION('',(0.,-1.,0.));
#2405=DIRECTION('center_axis',(0.,-1.,0.));
#2406=DIRECTION('ref_axis',(0.,0.,1.));
#2407=DIRECTION('center_axis',(0.,0.978147600733806,0.207911690817759));
#2408=DIRECTION('ref_axis',(0.,-0.207911690817759,0.978147600733806));
#2409=DIRECTION('center_axis',(0.,-0.811541913546029,-0.5842942089034));
#2410=DIRECTION('ref_axis',(0.,-0.5842942089034,0.811541913546029));
#2411=DIRECTION('',(0.,-1.,0.));
#2412=DIRECTION('',(0.,-1.,0.));
#2413=DIRECTION('center_axis',(0.,-1.,0.));
#2414=DIRECTION('ref_axis',(0.,0.,1.));
#2415=DIRECTION('center_axis',(0.,0.978147600733806,0.207911690817759));
#2416=DIRECTION('ref_axis',(0.,-0.207911690817759,0.978147600733806));
#2417=DIRECTION('',(0.,-1.,0.));
#2418=DIRECTION('',(0.,-1.,0.));
#2419=DIRECTION('center_axis',(0.,-0.811541913546029,-0.5842942089034));
#2420=DIRECTION('ref_axis',(0.,-0.5842942089034,0.811541913546029));
#2421=DIRECTION('center_axis',(-0.994206946103325,0.,0.107482781504297));
#2422=DIRECTION('ref_axis',(-0.107482781504297,0.,-0.994206946103325));
#2423=DIRECTION('',(0.,-1.,0.));
#2424=DIRECTION('',(0.105160285869614,-0.206758879790012,0.972724051262125));
#2425=DIRECTION('',(-0.0873993054910777,0.582058324791578,-0.808436434075369));
#2426=DIRECTION('center_axis',(0.,-1.,0.));
#2427=DIRECTION('ref_axis',(7.6571373978539E-16,0.,-1.));
#2428=DIRECTION('center_axis',(0.,0.978147600733806,0.207911690817759));
#2429=DIRECTION('ref_axis',(0.,-0.207911690817759,0.978147600733806));
#2430=DIRECTION('center_axis',(0.,-0.811541913546029,-0.5842942089034));
#2431=DIRECTION('ref_axis',(0.,-0.5842942089034,0.811541913546029));
#2432=DIRECTION('',(0.,-1.,0.));
#2433=DIRECTION('center_axis',(-0.994206946103325,0.,-0.107482781504297));
#2434=DIRECTION('ref_axis',(0.107482781504297,0.,-0.994206946103325));
#2435=DIRECTION('',(-0.105160285869614,-0.206758879790012,0.972724051262125));
#2436=DIRECTION('',(0.0873993054910777,0.582058324791578,-0.808436434075369));
#2437=DIRECTION('center_axis',(0.994206946103325,0.,0.107482781504297));
#2438=DIRECTION('ref_axis',(-0.107482781504297,0.,0.994206946103325));
#2439=DIRECTION('center_axis',(0.,-1.,0.));
#2440=DIRECTION('ref_axis',(0.,0.,1.));
#2441=DIRECTION('',(-1.,0.,0.));
#2442=DIRECTION('',(0.111883696952722,0.,0.99372130819269));
#2443=DIRECTION('',(-1.,0.,0.));
#2444=DIRECTION('center_axis',(0.,0.,1.));
#2445=DIRECTION('ref_axis',(-1.,0.,0.));
#2446=DIRECTION('',(-1.,0.,0.));
#2447=DIRECTION('',(0.,1.,0.));
#2448=DIRECTION('center_axis',(0.,-0.978147600733806,-0.207911690817759));
#2449=DIRECTION('ref_axis',(0.,-0.207911690817759,0.978147600733806));
#2450=DIRECTION('',(-1.,0.,0.));
#2451=DIRECTION('center_axis',(0.,0.978147600733806,0.207911690817759));
#2452=DIRECTION('ref_axis',(0.,-0.207911690817759,0.978147600733806));
#2453=DIRECTION('',(0.109468391364691,-0.206662199202023,0.97226920485687));
#2454=DIRECTION('',(-1.,0.,0.));
#2455=DIRECTION('center_axis',(-1.,0.,0.));
#2456=DIRECTION('ref_axis',(0.,-0.404767724305038,0.914419536843412));
#2457=DIRECTION('',(-1.,0.,0.));
#2458=DIRECTION('center_axis',(-1.,0.,0.));
#2459=DIRECTION('ref_axis',(0.,-0.40476772430504,0.914419536843411));
#2460=DIRECTION('',(-1.,0.,0.));
#2461=DIRECTION('center_axis',(-1.,0.,0.));
#2462=DIRECTION('ref_axis',(0.,0.,1.));
#2463=DIRECTION('center_axis',(0.,0.811541913546029,0.5842942089034));
#2464=DIRECTION('ref_axis',(0.,0.5842942089034,-0.811541913546029));
#2465=DIRECTION('center_axis',(0.,-0.811541913546029,-0.5842942089034));
#2466=DIRECTION('ref_axis',(-0.137420443729346,0.578750897214899,-0.803842659118176));
#2467=DIRECTION('center_axis',(0.,-0.811541913546029,-0.5842942089034));
#2468=DIRECTION('ref_axis',(0.,-0.5842942089034,0.811541913546029));
#2469=DIRECTION('center_axis',(0.,-0.811541913546029,-0.5842942089034));
#2470=DIRECTION('ref_axis',(-0.137420443729346,-0.578750897214899,0.803842659118176));
#2471=DIRECTION('center_axis',(0.,0.,1.));
#2472=DIRECTION('ref_axis',(-1.,0.,0.));
#2473=DIRECTION('',(0.,-1.,0.));
#2474=DIRECTION('center_axis',(0.,0.,-1.));
#2475=DIRECTION('ref_axis',(-1.,0.,0.));
#2476=DIRECTION('center_axis',(0.,0.,-1.));
#2477=DIRECTION('ref_axis',(-1.,0.,0.));
#2478=DIRECTION('center_axis',(-1.,0.,0.));
#2479=DIRECTION('ref_axis',(0.,0.,-1.));
#2480=DIRECTION('',(-1.,0.,0.));
#2481=DIRECTION('center_axis',(0.99372130819269,0.,-0.111883696952722));
#2482=DIRECTION('ref_axis',(-0.111883696952722,0.,-0.99372130819269));
#2483=DIRECTION('center_axis',(1.,0.,0.));
#2484=DIRECTION('ref_axis',(0.,0.,1.));
#2485=DIRECTION('',(0.,-1.,0.));
#2486=DIRECTION('center_axis',(0.,-1.,0.));
#2487=DIRECTION('ref_axis',(0.,0.,1.));
#2488=DIRECTION('',(0.,-1.,0.));
#2489=DIRECTION('',(0.,-1.,0.));
#2490=DIRECTION('center_axis',(0.0838731194178255,-0.675424884481499,0.732643518542461));
#2491=DIRECTION('ref_axis',(-0.993606933527829,-0.000929771706171516,0.112891085431926));
#2492=DIRECTION('center_axis',(-0.99372130819269,0.,0.111883696952722));
#2493=DIRECTION('ref_axis',(-0.111883696952722,0.,-0.99372130819269));
#2494=DIRECTION('',(-0.111883696952722,0.,-0.99372130819269));
#2495=DIRECTION('center_axis',(-0.111883696952722,0.,-0.99372130819269));
#2496=DIRECTION('ref_axis',(0.99372130819269,0.,-0.111883696952722));
#2497=DIRECTION('center_axis',(1.,0.,0.));
#2498=DIRECTION('ref_axis',(0.,0.,1.));
#2499=DIRECTION('center_axis',(-0.111883696952722,0.,0.99372130819269));
#2500=DIRECTION('ref_axis',(-0.99372130819269,0.,-0.111883696952722));
#3464=CARTESIAN_POINT('',(0.,0.,0.));
#3465=CARTESIAN_POINT('Origin',(0.03302,0.,-4.66590430475142E-19));
#3466=CARTESIAN_POINT('',(0.027604181732227,-0.00545787893630659,-0.00531751422345259));
#3467=CARTESIAN_POINT('',(0.0226758178125118,9.62593038363268E-18,0.00762));
#3468=CARTESIAN_POINT('Ctrl Pts',(0.027604181732227,-0.00545787893630659,
-0.00531751422345262));
#3469=CARTESIAN_POINT('Ctrl Pts',(0.0275279686032949,-0.00611737521333048,
-0.00464060943529688));
#3470=CARTESIAN_POINT('Ctrl Pts',(0.0274058826755258,-0.0066799041580939,
-0.00379613683788713));
#3471=CARTESIAN_POINT('Ctrl Pts',(0.0270288812884003,-0.00743795219517752,
-0.00194362990368062));
#3472=CARTESIAN_POINT('Ctrl Pts',(0.0267664171994647,-0.00762,-0.000931205111824686));
#3473=CARTESIAN_POINT('Ctrl Pts',(0.0261584464192118,-0.00762,0.000978832298277093));
#3474=CARTESIAN_POINT('Ctrl Pts',(0.0257672989424535,-0.00742146342376193,
0.00200253544380404));
#3475=CARTESIAN_POINT('Ctrl Pts',(0.0249302786493874,-0.00664164931271475,
0.00386998191769847));
#3476=CARTESIAN_POINT('Ctrl Pts',(0.0244863308943722,-0.00606132290844568,
0.00471498443683733));
#3477=CARTESIAN_POINT('Ctrl Pts',(0.0237267319642579,-0.0047360597713164,
0.00604024757396661));
#3478=CARTESIAN_POINT('Ctrl Pts',(0.023353947088258,-0.00390186974450739,
0.00662341729985035));
#3479=CARTESIAN_POINT('Ctrl Pts',(0.0228253280612608,-0.00203244645804173,
0.00741372953304487));
#3480=CARTESIAN_POINT('Ctrl Pts',(0.0226758178125118,-0.000995062388186708,
0.00762));
#3481=CARTESIAN_POINT('Ctrl Pts',(0.0226758178125118,1.66533453693773E-17,
0.00762));
#3482=CARTESIAN_POINT('',(0.027604181732227,0.00545787893630665,-0.00531751422345258));
#3483=CARTESIAN_POINT('Origin',(0.0270054795156059,0.,-4.66590430475142E-19));
#3484=CARTESIAN_POINT('Ctrl Pts',(0.0226758178125118,1.80411241501588E-17,
0.00762));
#3485=CARTESIAN_POINT('Ctrl Pts',(0.0226758178125118,0.000968408409381741,
0.00762));
#3486=CARTESIAN_POINT('Ctrl Pts',(0.0228174879353441,0.00198103471135963,
0.0074243825187784));
#3487=CARTESIAN_POINT('Ctrl Pts',(0.0233228057036299,0.00381368713962225,
0.00667096418394018));
#3488=CARTESIAN_POINT('Ctrl Pts',(0.0236805646112505,0.00463571714263501,
0.00611410121403885));
#3489=CARTESIAN_POINT('Ctrl Pts',(0.0244337098519972,0.00598793937687868,
0.00481301069798848));
#3490=CARTESIAN_POINT('Ctrl Pts',(0.0248888180929435,0.00659481223922085,
0.00395546133059954));
#3491=CARTESIAN_POINT('Ctrl Pts',(0.0257482260040042,0.0074113450160527,
0.00205163105595064));
#3492=CARTESIAN_POINT('Ctrl Pts',(0.0261504419883698,0.00762,0.00100397949753623));
#3493=CARTESIAN_POINT('Ctrl Pts',(0.0267667596758862,0.00762,-0.000932281056258697));
#3494=CARTESIAN_POINT('Ctrl Pts',(0.0270294385011349,0.00743753112566452,
-0.00194582582065931));
#3495=CARTESIAN_POINT('Ctrl Pts',(0.0274061392648596,0.00667871192581181,
-0.00379792191976084));
#3496=CARTESIAN_POINT('Ctrl Pts',(0.0275280372657644,0.00611678105529415,
-0.00464121927713181));
#3497=CARTESIAN_POINT('Ctrl Pts',(0.027604181732227,0.00545787893630661,
-0.00531751422345259));
#3498=CARTESIAN_POINT('',(0.0195416906937108,9.33180860950283E-19,0.00762));
#3499=CARTESIAN_POINT('',(0.03302,9.33180860950283E-19,0.00762));
#3500=CARTESIAN_POINT('',(0.0226351769200258,0.00396239491185587,-0.00650875));
#3501=CARTESIAN_POINT('Ctrl Pts',(0.0226351769200262,0.00396239491186084,
-0.00650874999999688));
#3502=CARTESIAN_POINT('Ctrl Pts',(0.0226703616592435,0.00449699874218484,
-0.00618329403731001));
#3503=CARTESIAN_POINT('Ctrl Pts',(0.0227049383031407,0.00498388799643907,
-0.00579469570810441));
#3504=CARTESIAN_POINT('Ctrl Pts',(0.022768434338136,0.00607818973523789,
-0.00469434328989012));
#3505=CARTESIAN_POINT('Ctrl Pts',(0.0227852939482288,0.00666267377651843,
-0.00383423955078307));
#3506=CARTESIAN_POINT('Ctrl Pts',(0.0226891534147118,0.00743351627485408,
-0.00195843047568892));
#3507=CARTESIAN_POINT('Ctrl Pts',(0.0225727993083733,0.00762,-0.000942950025364602));
#3508=CARTESIAN_POINT('Ctrl Pts',(0.022222087775008,0.00762,0.000991367009882884));
#3509=CARTESIAN_POINT('Ctrl Pts',(0.0219595192234926,0.00741593649953567,
0.00202962035276651));
#3510=CARTESIAN_POINT('Ctrl Pts',(0.0213461292163487,0.00661579385613863,
0.00391749182253754));
#3511=CARTESIAN_POINT('Ctrl Pts',(0.0209980046436713,0.00602056849457482,
0.00476834679472658));
#3512=CARTESIAN_POINT('Ctrl Pts',(0.0203927163583856,0.00467684447142528,
0.00608634155064048));
#3513=CARTESIAN_POINT('Ctrl Pts',(0.0200909975583043,0.00384158541585977,
0.00665672394664847));
#3514=CARTESIAN_POINT('Ctrl Pts',(0.0196624939401288,0.00198880319602538,
0.00742390702765397));
#3515=CARTESIAN_POINT('Ctrl Pts',(0.0195416906937108,0.000969608868230746,
0.00762));
#3516=CARTESIAN_POINT('Ctrl Pts',(0.0195416906937108,2.77555756156289E-19,
0.00762));
#3517=CARTESIAN_POINT('',(0.0226351769200258,-0.00396239491185566,-0.00650875));
#3518=CARTESIAN_POINT('Origin',(0.0233388317846976,0.,-4.66590430475142E-19));
#3519=CARTESIAN_POINT('Ctrl Pts',(0.0195416906937108,2.77555756156289E-19,
0.00762));
#3520=CARTESIAN_POINT('Ctrl Pts',(0.0195416906937108,-0.000969608868230745,
0.00762));
#3521=CARTESIAN_POINT('Ctrl Pts',(0.0196624939401288,-0.00198880319602538,
0.00742390702765397));
#3522=CARTESIAN_POINT('Ctrl Pts',(0.0200909975583043,-0.00384158541585977,
0.00665672394664847));
#3523=CARTESIAN_POINT('Ctrl Pts',(0.0203927163583856,-0.00467684447142528,
0.00608634155064048));
#3524=CARTESIAN_POINT('Ctrl Pts',(0.0209980046436713,-0.00602056849457482,
0.00476834679472658));
#3525=CARTESIAN_POINT('Ctrl Pts',(0.0213461292163487,-0.00661579385613863,
0.00391749182253753));
#3526=CARTESIAN_POINT('Ctrl Pts',(0.0219595192234926,-0.00741593649953567,
0.0020296203527665));
#3527=CARTESIAN_POINT('Ctrl Pts',(0.022222087775008,-0.00762000000000002,
0.000991367009882883));
#3528=CARTESIAN_POINT('Ctrl Pts',(0.0225727993083733,-0.00762000000000002,
-0.000942950025364605));
#3529=CARTESIAN_POINT('Ctrl Pts',(0.0226891534147118,-0.00743351627485408,
-0.00195843047568891));
#3530=CARTESIAN_POINT('Ctrl Pts',(0.0227852939482288,-0.00666267377651843,
-0.00383423955078307));
#3531=CARTESIAN_POINT('Ctrl Pts',(0.022768434338136,-0.00607818973523789,
-0.00469434328989012));
#3532=CARTESIAN_POINT('Ctrl Pts',(0.0227049383031407,-0.00498388799643903,
-0.00579469570810445));
#3533=CARTESIAN_POINT('Ctrl Pts',(0.0226703616592435,-0.00449699874218474,
-0.00618329403731008));
#3534=CARTESIAN_POINT('Ctrl Pts',(0.0226351769200262,-0.00396239491186069,
-0.00650874999999697));
#3535=CARTESIAN_POINT('Origin',(0.019796125,0.142748,0.0130716462696265));
#3536=CARTESIAN_POINT('',(0.019796125,0.0102506251722644,0.0110620425392529));
#3537=CARTESIAN_POINT('',(0.019796125,-0.0102506251722643,0.0110620425392529));
#3538=CARTESIAN_POINT('',(0.019796125,0.142748,0.0110620425392529));
#3539=CARTESIAN_POINT('Origin',(0.019796125,5.89805981832114E-17,2.47198095326695E-17));
#3540=CARTESIAN_POINT('Origin',(2.94902990916057E-17,0.142748,-0.0084254861247228));
#3541=CARTESIAN_POINT('',(0.0274949578025845,0.0217988744690902,-0.00446598692924329));
#3542=CARTESIAN_POINT('',(0.0217835558367569,0.012239066483666,0.0088118870380244));
#3543=CARTESIAN_POINT('Origin',(2.94902990916057E-17,0.0246496359780892,
-0.0084254861247228));
#3544=CARTESIAN_POINT('Ctrl Pts',(0.019796125,0.0102506251722644,0.0110620425392529));
#3545=CARTESIAN_POINT('Ctrl Pts',(0.0199250556804199,0.0103919650352694,
0.0109310701666171));
#3546=CARTESIAN_POINT('Ctrl Pts',(0.020053197009147,0.0105298129337859,
0.0107982953537534));
#3547=CARTESIAN_POINT('Ctrl Pts',(0.0201801831206385,0.0106640541437697,
0.0106640541437696));
#3548=CARTESIAN_POINT('Ctrl Pts',(0.0207051784182023,0.0112190440017391,
0.0101090642858003));
#3549=CARTESIAN_POINT('Ctrl Pts',(0.0212473394853561,0.0117511804678545,
0.00948952502387266));
#3550=CARTESIAN_POINT('Ctrl Pts',(0.0217835558367568,0.0122390664836661,
0.00881188703802442));
#3551=CARTESIAN_POINT('',(0.0272702604802117,-0.0147516885035667,-0.00313556818714528));
#3552=CARTESIAN_POINT('Ctrl Pts',(0.0272702604802117,-0.0147516885035667,
-0.00313556818714528));
#3553=CARTESIAN_POINT('Ctrl Pts',(0.0272495688109927,-0.0147743615770061,
-0.00302889976316783));
#3554=CARTESIAN_POINT('Ctrl Pts',(0.0272282288068284,-0.0147958237878268,
-0.00292223786676003));
#3555=CARTESIAN_POINT('Ctrl Pts',(0.027009028365588,-0.0149978474224452,
-0.0018591751296926));
#3556=CARTESIAN_POINT('Ctrl Pts',(0.0267588953224807,-0.0150812499999999,
-0.000907573932662182));
#3557=CARTESIAN_POINT('Ctrl Pts',(0.0261291401823591,-0.0150812499999999,
0.00107090252690661));
#3558=CARTESIAN_POINT('Ctrl Pts',(0.025713893024289,-0.0149657875440865,
0.00214629933068523));
#3559=CARTESIAN_POINT('Ctrl Pts',(0.0247544184553272,-0.0145148320065805,
0.00423096318224476));
#3560=CARTESIAN_POINT('Ctrl Pts',(0.0242102662610114,-0.0141796498547937,
0.00524033209572036));
#3561=CARTESIAN_POINT('Ctrl Pts',(0.0224519953219796,-0.0129007914315354,
0.008082788964929));
#3562=CARTESIAN_POINT('Ctrl Pts',(0.0211034211368484,-0.0116760800285812,
0.00972638603161029));
#3563=CARTESIAN_POINT('Ctrl Pts',(0.0198342735534848,-0.0102923878241089,
0.0110232329058798));
#3564=CARTESIAN_POINT('Ctrl Pts',(0.0198152109382652,-0.0102715480735547,
0.0110426543640688));
#3565=CARTESIAN_POINT('Ctrl Pts',(0.019796125,-0.0102506251722643,0.0110620425392529));
#3566=CARTESIAN_POINT('',(0.027604181732227,-0.0142879015563397,-0.00531751422345259));
#3567=CARTESIAN_POINT('Origin',(2.94902990916057E-17,-0.0136272817352386,
-0.0084254861247228));
#3568=CARTESIAN_POINT('',(0.027604181732227,0.142748,-0.00531751422345259));
#3569=CARTESIAN_POINT('',(0.027604181732227,0.0208616467784906,-0.00531751422345259));
#3570=CARTESIAN_POINT('',(0.027604181732227,0.142748,-0.00531751422345259));
#3571=CARTESIAN_POINT('Origin',(-0.0328868893532025,0.020918252442196,-0.0121903564161812));
#3572=CARTESIAN_POINT('Origin',(0.0303120908661135,0.142748,-0.0293684446117263));
#3573=CARTESIAN_POINT('',(0.0325400145420211,-0.00496968603632477,-0.0491562715255243));
#3574=CARTESIAN_POINT('',(0.0299860624391297,-0.00979121809375477,-0.0264727466343235));
#3575=CARTESIAN_POINT('',(0.0325400145420211,-0.009525,-0.0491562715255243));
#3576=CARTESIAN_POINT('',(0.0325400145420211,-0.00724734301816237,-0.0491562715255243));
#3577=CARTESIAN_POINT('',(0.03302,-0.009525,-0.053419375));
#3578=CARTESIAN_POINT('',(0.0327830114907868,-0.009525,-0.0513145059456507));
#3579=CARTESIAN_POINT('',(0.03302,0.0208616467784906,-0.053419375));
#3580=CARTESIAN_POINT('',(0.03302,0.022225,-0.053419375));
#3581=CARTESIAN_POINT('',(0.0303120908661135,0.0208616467784906,-0.0293684446117263));
#3582=CARTESIAN_POINT('Origin',(-0.017018,0.142748,0.0130716462696265));
#3583=CARTESIAN_POINT('',(-0.017018,0.0102506251722644,0.0110620425392529));
#3584=CARTESIAN_POINT('',(-0.017018,-0.0102506251722643,0.0110620425392529));
#3585=CARTESIAN_POINT('',(-0.017018,0.142748,0.0110620425392529));
#3586=CARTESIAN_POINT('Origin',(-0.017018,5.89805981832114E-17,2.47198095326695E-17));
#3587=CARTESIAN_POINT('Origin',(0.017018,0.142748,0.0130716462696265));
#3588=CARTESIAN_POINT('',(0.017018,-0.0102506251722643,0.0110620425392529));
#3589=CARTESIAN_POINT('',(0.017018,0.0102506251722644,0.0110620425392529));
#3590=CARTESIAN_POINT('Origin',(0.017018,5.89805981832114E-17,2.47198095326695E-17));
#3591=CARTESIAN_POINT('',(0.017018,0.142748,0.0110620425392529));
#3592=CARTESIAN_POINT('Origin',(-5.20417042793042E-18,0.142748,-0.0040616822293093));
#3593=CARTESIAN_POINT('',(0.0227482238351949,-0.0147516885035667,-0.00313556818714528));
#3594=CARTESIAN_POINT('',(0.0226351769200258,-0.0140346965755384,-0.00650875));
#3595=CARTESIAN_POINT('Origin',(-5.20417042793042E-18,-0.01455483688705,
-0.0040616822293093));
#3596=CARTESIAN_POINT('Ctrl Pts',(0.0227482238351949,-0.0147516885035667,
-0.00313556818714527));
#3597=CARTESIAN_POINT('Ctrl Pts',(0.0227446067595775,-0.0147705734226378,
-0.00304672162826799));
#3598=CARTESIAN_POINT('Ctrl Pts',(0.0227404659003224,-0.0147886314076116,
-0.00295781815060928));
#3599=CARTESIAN_POINT('Ctrl Pts',(0.0226851188015466,-0.0149930494779853,
-0.00190284970904404));
#3600=CARTESIAN_POINT('Ctrl Pts',(0.0225710627210582,-0.0150812499999999,
-0.000933372038593934));
#3601=CARTESIAN_POINT('Ctrl Pts',(0.0222119151141167,-0.0150812499999999,
0.00104747338045759));
#3602=CARTESIAN_POINT('Ctrl Pts',(0.0219431733917285,-0.0149706590076676,
0.00210320147053684));
#3603=CARTESIAN_POINT('Ctrl Pts',(0.0212601083230291,-0.0145354311779761,
0.00415515679714474));
#3604=CARTESIAN_POINT('Ctrl Pts',(0.0208459021049179,-0.0142110577693777,
0.00515147888694799));
#3605=CARTESIAN_POINT('Ctrl Pts',(0.0194466634913425,-0.0129714177672581,
0.00796100440593939));
#3606=CARTESIAN_POINT('Ctrl Pts',(0.0182957954663637,-0.0117801714359752,
0.0095915927647639));
#3607=CARTESIAN_POINT('Ctrl Pts',(0.0171380411001156,-0.0103958203260114,
0.0109261520357052));
#3608=CARTESIAN_POINT('Ctrl Pts',(0.0170781669004994,-0.0103236873082037,
0.0109943396202718));
#3609=CARTESIAN_POINT('Ctrl Pts',(0.017018,-0.0102506251722643,0.0110620425392529));
#3610=CARTESIAN_POINT('',(0.0187779282455329,0.012239066483666,0.0088118870380244));
#3611=CARTESIAN_POINT('Ctrl Pts',(0.017018,0.0102506251722644,0.0110620425392529));
#3612=CARTESIAN_POINT('Ctrl Pts',(0.0170781669004994,0.0103236873082038,
0.0109943396202718));
#3613=CARTESIAN_POINT('Ctrl Pts',(0.0171380411001156,0.0103958203260115,
0.0109261520357052));
#3614=CARTESIAN_POINT('Ctrl Pts',(0.017721633324578,0.011093633754536,0.0102534373076843));
#3615=CARTESIAN_POINT('Ctrl Pts',(0.018259156437714,0.0116942557001332,
0.00956858936204477));
#3616=CARTESIAN_POINT('Ctrl Pts',(0.0187779282455329,0.0122390664836661,
0.00881188703802446));
#3617=CARTESIAN_POINT('',(0.0226351769200258,0.0232696236842349,-0.00650875));
#3618=CARTESIAN_POINT('Origin',(-5.20417042793042E-18,0.0215077830407108,
-0.0040616822293093));
#3619=CARTESIAN_POINT('',(0.0226351769200258,0.142748,-0.00650875));
#3620=CARTESIAN_POINT('',(0.0226351769200258,0.142748,-0.00650875));
#3621=CARTESIAN_POINT('Origin',(2.42861286636753E-17,0.142748,-0.00406168222930931));
#3622=CARTESIAN_POINT('',(-0.0226351769200258,-0.0140346965755384,-0.00650875));
#3623=CARTESIAN_POINT('',(-0.0227482238351949,-0.0147516885035667,-0.00313556818714528));
#3624=CARTESIAN_POINT('Origin',(2.42861286636753E-17,-0.01455483688705,
-0.00406168222930931));
#3625=CARTESIAN_POINT('',(-0.0226351769200258,-0.00396239491185574,-0.00650875));
#3626=CARTESIAN_POINT('',(-0.0226351769200258,0.142748,-0.00650875));
#3627=CARTESIAN_POINT('',(-0.0195416906937107,9.33180860950283E-19,0.00762));
#3628=CARTESIAN_POINT('Ctrl Pts',(-0.0226351769200261,-0.00396239491186075,
-0.00650874999999693));
#3629=CARTESIAN_POINT('Ctrl Pts',(-0.0226703616592435,-0.00449699874218478,
-0.00618329403731005));
#3630=CARTESIAN_POINT('Ctrl Pts',(-0.0227049383031407,-0.00498388799643905,
-0.00579469570810443));
#3631=CARTESIAN_POINT('Ctrl Pts',(-0.022768434338136,-0.00607818973523789,
-0.00469434328989012));
#3632=CARTESIAN_POINT('Ctrl Pts',(-0.0227852939482288,-0.00666267377651843,
-0.00383423955078307));
#3633=CARTESIAN_POINT('Ctrl Pts',(-0.0226891534147118,-0.00743351627485408,
-0.00195843047568891));
#3634=CARTESIAN_POINT('Ctrl Pts',(-0.0225727993083733,-0.00762000000000002,
-0.000942950025364604));
#3635=CARTESIAN_POINT('Ctrl Pts',(-0.0222220877750079,-0.00762000000000002,
0.000991367009882883));
#3636=CARTESIAN_POINT('Ctrl Pts',(-0.0219595192234926,-0.00741593649953567,
0.0020296203527665));
#3637=CARTESIAN_POINT('Ctrl Pts',(-0.0213461292163486,-0.00661579385613864,
0.00391749182253753));
#3638=CARTESIAN_POINT('Ctrl Pts',(-0.0209980046436713,-0.00602056849457482,
0.00476834679472658));
#3639=CARTESIAN_POINT('Ctrl Pts',(-0.0203927163583856,-0.00467684447142528,
0.00608634155064047));
#3640=CARTESIAN_POINT('Ctrl Pts',(-0.0200909975583043,-0.00384158541585977,
0.00665672394664846));
#3641=CARTESIAN_POINT('Ctrl Pts',(-0.0196624939401288,-0.00198880319602538,
0.00742390702765397));
#3642=CARTESIAN_POINT('Ctrl Pts',(-0.0195416906937107,-0.000969608868230746,
0.00762));
#3643=CARTESIAN_POINT('Ctrl Pts',(-0.0195416906937107,-2.77555756156289E-19,
0.00762));
#3644=CARTESIAN_POINT('',(-0.0226351769200258,0.0039623949118558,-0.00650875));
#3645=CARTESIAN_POINT('Ctrl Pts',(-0.0195416906937107,0.,0.00762));
#3646=CARTESIAN_POINT('Ctrl Pts',(-0.0195416906937107,0.000969608868230746,
0.00762));
#3647=CARTESIAN_POINT('Ctrl Pts',(-0.0196624939401288,0.00198880319602538,
0.00742390702765397));
#3648=CARTESIAN_POINT('Ctrl Pts',(-0.0200909975583043,0.00384158541585977,
0.00665672394664847));
#3649=CARTESIAN_POINT('Ctrl Pts',(-0.0203927163583856,0.00467684447142528,
0.00608634155064048));
#3650=CARTESIAN_POINT('Ctrl Pts',(-0.0209980046436713,0.00602056849457482,
0.00476834679472658));
#3651=CARTESIAN_POINT('Ctrl Pts',(-0.0213461292163486,0.00661579385613863,
0.00391749182253754));
#3652=CARTESIAN_POINT('Ctrl Pts',(-0.0219595192234926,0.00741593649953567,
0.00202962035276651));
#3653=CARTESIAN_POINT('Ctrl Pts',(-0.0222220877750079,0.00762,0.000991367009882883));
#3654=CARTESIAN_POINT('Ctrl Pts',(-0.0225727993083733,0.00762,-0.000942950025364602));
#3655=CARTESIAN_POINT('Ctrl Pts',(-0.0226891534147118,0.00743351627485408,
-0.00195843047568892));
#3656=CARTESIAN_POINT('Ctrl Pts',(-0.0227852939482288,0.00666267377651843,
-0.00383423955078308));
#3657=CARTESIAN_POINT('Ctrl Pts',(-0.022768434338136,0.00607818973523789,
-0.00469434328989012));
#3658=CARTESIAN_POINT('Ctrl Pts',(-0.0227049383031407,0.00498388799643906,
-0.00579469570810442));
#3659=CARTESIAN_POINT('Ctrl Pts',(-0.0226703616592435,0.00449699874218481,
-0.00618329403731003));
#3660=CARTESIAN_POINT('Ctrl Pts',(-0.0226351769200261,0.00396239491186079,
-0.00650874999999691));
#3661=CARTESIAN_POINT('',(-0.0226351769200258,0.0232696236842349,-0.00650875));
#3662=CARTESIAN_POINT('',(-0.0226351769200258,0.142748,-0.00650875));
#3663=CARTESIAN_POINT('',(-0.0187779282455329,0.012239066483666,0.0088118870380244));
#3664=CARTESIAN_POINT('Origin',(2.42861286636753E-17,0.0215077830407108,
-0.00406168222930931));
#3665=CARTESIAN_POINT('Ctrl Pts',(-0.0187779282455329,0.0122390664836661,
0.00881188703802446));
#3666=CARTESIAN_POINT('Ctrl Pts',(-0.0183124690330524,0.0117502442415317,
0.00949082537374769));
#3667=CARTESIAN_POINT('Ctrl Pts',(-0.017832992880629,0.0112176146967558,
0.0101104935907835));
#3668=CARTESIAN_POINT('Ctrl Pts',(-0.0172495397298473,0.0105296488003802,
0.0107984594871591));
#3669=CARTESIAN_POINT('Ctrl Pts',(-0.0171342563174104,0.0103917980562914,
0.0109312248974374));
#3670=CARTESIAN_POINT('Ctrl Pts',(-0.017018,0.0102506251722644,0.0110620425392529));
#3671=CARTESIAN_POINT('Ctrl Pts',(-0.017018,-0.0102506251722643,0.0110620425392529));
#3672=CARTESIAN_POINT('Ctrl Pts',(-0.0170781669004994,-0.0103236873082037,
0.0109943396202718));
#3673=CARTESIAN_POINT('Ctrl Pts',(-0.0171380411001156,-0.0103958203260114,
0.0109261520357052));
#3674=CARTESIAN_POINT('Ctrl Pts',(-0.0182957954663637,-0.0117801714359752,
0.00959159276476389));
#3675=CARTESIAN_POINT('Ctrl Pts',(-0.0194466634913425,-0.0129714177672581,
0.00796100440593937));
#3676=CARTESIAN_POINT('Ctrl Pts',(-0.0208459021049179,-0.0142110577693777,
0.00515147888694798));
#3677=CARTESIAN_POINT('Ctrl Pts',(-0.0212601083230291,-0.0145354311779761,
0.00415515679714473));
#3678=CARTESIAN_POINT('Ctrl Pts',(-0.0219431733917285,-0.0149706590076676,
0.00210320147053683));
#3679=CARTESIAN_POINT('Ctrl Pts',(-0.0222119151141167,-0.0150812499999999,
0.00104747338045759));
#3680=CARTESIAN_POINT('Ctrl Pts',(-0.0225710627210582,-0.0150812499999999,
-0.000933372038593937));
#3681=CARTESIAN_POINT('Ctrl Pts',(-0.0226851188015466,-0.0149930494779853,
-0.00190284970904404));
#3682=CARTESIAN_POINT('Ctrl Pts',(-0.0227404659003224,-0.0147886314076116,
-0.00295781815060928));
#3683=CARTESIAN_POINT('Ctrl Pts',(-0.0227446067595775,-0.0147705734226378,
-0.003046721628268));
#3684=CARTESIAN_POINT('Ctrl Pts',(-0.0227482238351949,-0.0147516885035667,
-0.00313556818714527));
#3685=CARTESIAN_POINT('Origin',(0.0214187310324227,0.142748,-0.0177607750600836));
#3686=CARTESIAN_POINT('',(0.0202022851448196,0.0394720969546926,-0.0290128001201673));
#3687=CARTESIAN_POINT('',(0.0202022851448196,-0.00925131305834584,-0.0290128001201673));
#3688=CARTESIAN_POINT('',(0.0202022851448196,0.142748,-0.0290128001201673));
#3689=CARTESIAN_POINT('',(0.0206505404826075,-0.0101326416961916,-0.0248664748742124));
#3690=CARTESIAN_POINT('',(0.0212486442437504,0.0325035973672875,-0.019334063956889));
#3691=CARTESIAN_POINT('Origin',(-2.20309881449055E-16,0.142748,-0.02682875));
#3692=CARTESIAN_POINT('',(-0.0202022851448196,-0.00925131305834583,-0.0290128001201673));
#3693=CARTESIAN_POINT('Origin',(-2.20309881449055E-16,-0.00971554724240362,
-0.02682875));
#3694=CARTESIAN_POINT('',(-0.0202022851448196,0.0394720969546926,-0.0290128001201673));
#3695=CARTESIAN_POINT('Origin',(-2.20309881449055E-16,0.0378996238441018,
-0.02682875));
#3696=CARTESIAN_POINT('',(-0.0202022851448196,0.142748,-0.0290128001201673));
#3697=CARTESIAN_POINT('Origin',(-0.0214187310324227,0.142748,-0.0177607750600836));
#3698=CARTESIAN_POINT('',(-0.0199202248773828,-0.00869674567155872,-0.0316218345457809));
#3699=CARTESIAN_POINT('',(-0.020744188550585,0.0358631507875988,-0.0240002378977473));
#3700=CARTESIAN_POINT('Origin',(-0.0233388317846976,0.,-4.66590430475142E-19));
#3701=CARTESIAN_POINT('Origin',(0.03302,-0.009525,-0.0512878232627621));
#3702=CARTESIAN_POINT('',(-0.032540014542021,-0.009525,-0.0491562715255243));
#3703=CARTESIAN_POINT('',(0.03302,-0.009525,-0.0491562715255243));
#3704=CARTESIAN_POINT('',(-0.03302,-0.009525,-0.053419375));
#3705=CARTESIAN_POINT('',(-0.0319563253038297,-0.009525,-0.0439720985928172));
#3706=CARTESIAN_POINT('',(0.03302,-0.009525,-0.053419375));
#3707=CARTESIAN_POINT('Origin',(0.03302,-0.00724734301816237,-0.0491562715255243));
#3708=CARTESIAN_POINT('',(-0.0325400145420211,-0.00496968603632477,-0.0491562715255243));
#3709=CARTESIAN_POINT('',(0.03302,-0.00496968603632477,-0.0491562715255243));
#3710=CARTESIAN_POINT('',(-0.032540014542021,-0.00724734301816237,-0.0491562715255243));
#3711=CARTESIAN_POINT('Origin',(0.03302,-0.00986068726994574,-0.0261459198563348));
#3712=CARTESIAN_POINT('',(-0.0272702604802117,-0.0147516885035667,-0.00313556818714528));
#3713=CARTESIAN_POINT('',(0.03302,-0.0147516885035667,-0.0031355681871453));
#3714=CARTESIAN_POINT('',(-0.027604181732227,-0.0142879015563397,-0.00531751422345259));
#3715=CARTESIAN_POINT('Origin',(2.25514051876985E-17,-0.0136272817352386,
-0.0084254861247228));
#3716=CARTESIAN_POINT('',(-0.0291946834112552,-0.0112852395940622,-0.0194439280997692));
#3717=CARTESIAN_POINT('',(0.03302,-0.0147516885035667,-0.0031355681871453));
#3718=CARTESIAN_POINT('Origin',(0.03302,5.89805981832114E-17,2.47198095326695E-17));
#3719=CARTESIAN_POINT('',(0.03302,0.012239066483666,0.0088118870380244));
#3720=CARTESIAN_POINT('Origin',(0.03302,5.89805981832114E-17,2.47198095326695E-17));
#3721=CARTESIAN_POINT('',(-0.0217835558367568,0.012239066483666,0.0088118870380244));
#3722=CARTESIAN_POINT('',(0.03302,0.012239066483666,0.0088118870380244));
#3723=CARTESIAN_POINT('',(-0.019796125,0.0102506251722644,0.0110620425392529));
#3724=CARTESIAN_POINT('Ctrl Pts',(-0.0217835558367568,0.0122390664836661,
0.00881188703802445));
#3725=CARTESIAN_POINT('Ctrl Pts',(-0.0212473394853562,0.0117511804678545,
0.00948952502387266));
#3726=CARTESIAN_POINT('Ctrl Pts',(-0.0207051784182024,0.0112190440017391,
0.0101090642858003));
#3727=CARTESIAN_POINT('Ctrl Pts',(-0.0201801831206385,0.0106640541437697,
0.0106640541437697));
#3728=CARTESIAN_POINT('Ctrl Pts',(-0.020053197009147,0.0105298129337859,
0.0107982953537535));
#3729=CARTESIAN_POINT('Ctrl Pts',(-0.01992505568042,0.0103919650352694,
0.0109310701666172));
#3730=CARTESIAN_POINT('Ctrl Pts',(-0.019796125,0.0102506251722644,0.0110620425392529));
#3731=CARTESIAN_POINT('',(-0.019796125,-0.0102506251722643,0.0110620425392529));
#3732=CARTESIAN_POINT('Origin',(-0.019796125,5.89805981832114E-17,2.47198095326695E-17));
#3733=CARTESIAN_POINT('Ctrl Pts',(-0.019796125,-0.0102506251722643,0.0110620425392529));
#3734=CARTESIAN_POINT('Ctrl Pts',(-0.0198152109382653,-0.0102715480735547,
0.0110426543640688));
#3735=CARTESIAN_POINT('Ctrl Pts',(-0.0198342735534848,-0.0102923878241089,
0.0110232329058798));
#3736=CARTESIAN_POINT('Ctrl Pts',(-0.0211034211368485,-0.0116760800285813,
0.00972638603161028));
#3737=CARTESIAN_POINT('Ctrl Pts',(-0.0224519953219796,-0.0129007914315354,
0.00808278896492899));
#3738=CARTESIAN_POINT('Ctrl Pts',(-0.0242102662610114,-0.0141796498547937,
0.00524033209572035));
#3739=CARTESIAN_POINT('Ctrl Pts',(-0.0247544184553273,-0.0145148320065805,
0.00423096318224475));
#3740=CARTESIAN_POINT('Ctrl Pts',(-0.025713893024289,-0.0149657875440865,
0.00214629933068522));
#3741=CARTESIAN_POINT('Ctrl Pts',(-0.0261291401823591,-0.0150812499999999,
0.0010709025269066));
#3742=CARTESIAN_POINT('Ctrl Pts',(-0.0267588953224807,-0.0150812499999999,
-0.000907573932662187));
#3743=CARTESIAN_POINT('Ctrl Pts',(-0.027009028365588,-0.0149978474224452,
-0.0018591751296926));
#3744=CARTESIAN_POINT('Ctrl Pts',(-0.0272282288068284,-0.0147958237878268,
-0.00292223786676003));
#3745=CARTESIAN_POINT('Ctrl Pts',(-0.0272495688109927,-0.0147743615770061,
-0.00302889976316783));
#3746=CARTESIAN_POINT('Ctrl Pts',(-0.0272702604802117,-0.0147516885035667,
-0.00313556818714527));
#3747=CARTESIAN_POINT('Origin',(0.03302,0.033107033241833,-0.0201721922437499));
#3748=CARTESIAN_POINT('',(-0.0274949578025847,0.0217988744690917,-0.00446598692924536));
#3749=CARTESIAN_POINT('',(1.03779831950312E-15,0.0539658339565387,-0.0491435405616761));
#3750=CARTESIAN_POINT('Origin',(0.00596083144644427,0.0208616467784906,
-0.00316424622761118));
#3751=CARTESIAN_POINT('Origin',(2.25514051876985E-17,0.0246496359780892,
-0.0084254861247228));
#3752=CARTESIAN_POINT('Origin',(-0.00596083144644428,0.0208616467784906,
-0.00316424622761117));
#3753=CARTESIAN_POINT('Origin',(0.03302,0.022225,-0.053419375));
#3754=CARTESIAN_POINT('',(-0.03302,0.0208616467784906,-0.053419375));
#3755=CARTESIAN_POINT('',(-0.03302,0.022225,-0.053419375));
#3756=CARTESIAN_POINT('',(1.4662354446901E-13,0.0539736348755679,-0.053419375));
#3757=CARTESIAN_POINT('Origin',(0.000302575402688698,0.0208616467784906,
-0.053419375));
#3758=CARTESIAN_POINT('Origin',(-0.000302575402688701,0.0208616467784906,
-0.053419375));
#3759=CARTESIAN_POINT('Origin',(0.03302,0.,-4.66590430475142E-19));
#3760=CARTESIAN_POINT('',(-0.0226758178125118,1.89034674318853E-19,0.00762));
#3761=CARTESIAN_POINT('',(0.03302,9.33180860950283E-19,0.00762));
#3762=CARTESIAN_POINT('',(-0.027604181732227,0.00545787893630664,-0.00531751422345259));
#3763=CARTESIAN_POINT('Ctrl Pts',(-0.027604181732227,0.00545787893630661,
-0.0053175142234526));
#3764=CARTESIAN_POINT('Ctrl Pts',(-0.0275280372657645,0.00611678105529414,
-0.00464121927713182));
#3765=CARTESIAN_POINT('Ctrl Pts',(-0.0274061392648596,0.00667871192581181,
-0.00379792191976086));
#3766=CARTESIAN_POINT('Ctrl Pts',(-0.0270294385011349,0.00743753112566452,
-0.00194582582065932));
#3767=CARTESIAN_POINT('Ctrl Pts',(-0.0267667596758862,0.00761999999999999,
-0.000932281056258699));
#3768=CARTESIAN_POINT('Ctrl Pts',(-0.0261504419883699,0.00761999999999999,
0.00100397949753623));
#3769=CARTESIAN_POINT('Ctrl Pts',(-0.0257482260040043,0.0074113450160527,
0.00205163105595065));
#3770=CARTESIAN_POINT('Ctrl Pts',(-0.0248888180929436,0.00659481223922084,
0.00395546133059956));
#3771=CARTESIAN_POINT('Ctrl Pts',(-0.0244337098519972,0.00598793937687863,
0.00481301069798849));
#3772=CARTESIAN_POINT('Ctrl Pts',(-0.0236805646112506,0.00463571714263495,
0.00611410121403885));
#3773=CARTESIAN_POINT('Ctrl Pts',(-0.02332280570363,0.00381368713962221,
0.0066709641839402));
#3774=CARTESIAN_POINT('Ctrl Pts',(-0.0228174879353442,0.0019810347113596,
0.00742438251877841));
#3775=CARTESIAN_POINT('Ctrl Pts',(-0.0226758178125118,0.000968408409381716,
0.00762));
#3776=CARTESIAN_POINT('Ctrl Pts',(-0.0226758178125118,8.32667268468867E-19,
0.00762));
#3777=CARTESIAN_POINT('',(-0.027604181732227,-0.00545787893630657,-0.00531751422345261));
#3778=CARTESIAN_POINT('Origin',(-0.0270054795156059,0.,-4.66590430475142E-19));
#3779=CARTESIAN_POINT('Ctrl Pts',(-0.0226758178125118,-5.55111512312578E-19,
0.00762));
#3780=CARTESIAN_POINT('Ctrl Pts',(-0.0226758178125118,-0.000968408409381723,
0.00762));
#3781=CARTESIAN_POINT('Ctrl Pts',(-0.0228174879353442,-0.00198103471135961,
0.00742438251877841));
#3782=CARTESIAN_POINT('Ctrl Pts',(-0.02332280570363,-0.00381368713962224,
0.00667096418394019));
#3783=CARTESIAN_POINT('Ctrl Pts',(-0.0236805646112506,-0.00463571714263499,
0.00611410121403885));
#3784=CARTESIAN_POINT('Ctrl Pts',(-0.0244337098519972,-0.00598793937687866,
0.00481301069798848));
#3785=CARTESIAN_POINT('Ctrl Pts',(-0.0248888180929436,-0.00659481223922085,
0.00395546133059954));
#3786=CARTESIAN_POINT('Ctrl Pts',(-0.0257482260040043,-0.0074113450160527,
0.00205163105595064));
#3787=CARTESIAN_POINT('Ctrl Pts',(-0.0261504419883699,-0.00762000000000002,
0.00100397949753623));
#3788=CARTESIAN_POINT('Ctrl Pts',(-0.0267667596758862,-0.00762000000000002,
-0.000932281056258699));
#3789=CARTESIAN_POINT('Ctrl Pts',(-0.0270294385011349,-0.00743753112566452,
-0.00194582582065931));
#3790=CARTESIAN_POINT('Ctrl Pts',(-0.0274061392648597,-0.0066787119258118,
-0.00379792191976087));
#3791=CARTESIAN_POINT('Ctrl Pts',(-0.0275280372657645,-0.00611678105529412,
-0.00464121927713185));
#3792=CARTESIAN_POINT('Ctrl Pts',(-0.027604181732227,-0.00545787893630657,
-0.00531751422345264));
#3793=CARTESIAN_POINT('Origin',(-0.019796125,0.142748,0.0130716462696265));
#3794=CARTESIAN_POINT('',(-0.019796125,0.142748,0.0110620425392529));
#3795=CARTESIAN_POINT('Origin',(2.25514051876985E-17,0.142748,-0.0084254861247228));
#3796=CARTESIAN_POINT('',(-0.027604181732227,0.0208616467784906,-0.00531751422345259));
#3797=CARTESIAN_POINT('',(-0.027604181732227,0.142748,-0.00531751422345259));
#3798=CARTESIAN_POINT('',(-0.027604181732227,0.142748,-0.00531751422345259));
#3799=CARTESIAN_POINT('Origin',(0.0328868894519471,0.0209182515429762,-0.012190355439119));
#3800=CARTESIAN_POINT('Origin',(-0.0303120908661135,0.142748,-0.0293684446117263));
#3801=CARTESIAN_POINT('',(-0.0303120908661135,0.0208616467784906,-0.0293684446117263));
#3802=CARTESIAN_POINT('Origin',(0.000949119378095248,0.0208616467784906,
-0.047676942969741));
#3803=CARTESIAN_POINT('Origin',(-2.00577401909819E-18,0.0208616467784906,
-0.0561067694388323));
#3804=CARTESIAN_POINT('Origin',(-0.000122433191138131,0.0208616467784906,
-0.0550193503225745));
#3823=UNCERTAINTY_MEASURE_WITH_UNIT(LENGTH_MEASURE(1.E-5),#3833,
'DISTANCE_ACCURACY_VALUE',
'Maximum model space distance between geometric entities at asserted c
onnectivities');
#3824=UNCERTAINTY_MEASURE_WITH_UNIT(LENGTH_MEASURE(1.E-5),#3833,
'DISTANCE_ACCURACY_VALUE',
'Maximum model space distance between geometric entities at asserted c
onnectivities');
#3831=(
GEOMETRIC_REPRESENTATION_CONTEXT(3)
GLOBAL_UNCERTAINTY_ASSIGNED_CONTEXT((#3823))
GLOBAL_UNIT_ASSIGNED_CONTEXT((#3833,#3834,#3835))
REPRESENTATION_CONTEXT('','3D')
);
#3832=(
GEOMETRIC_REPRESENTATION_CONTEXT(3)
GLOBAL_UNCERTAINTY_ASSIGNED_CONTEXT((#3824))
GLOBAL_UNIT_ASSIGNED_CONTEXT((#3833,#3834,#3835))
REPRESENTATION_CONTEXT('','3D')
);
#3833=(
LENGTH_UNIT()
NAMED_UNIT(*)
SI_UNIT($,.METRE.)
);
#3834=(
NAMED_UNIT(*)
PLANE_ANGLE_UNIT()
SI_UNIT($,.RADIAN.)
);
#3835=(
NAMED_UNIT(*)
SI_UNIT($,.STERADIAN.)
SOLID_ANGLE_UNIT()
);
#3842=SHAPE_DEFINITION_REPRESENTATION(#3849,#3868);
#3849=PRODUCT_DEFINITION_SHAPE('',$,#3876);
#3868=SHAPE_REPRESENTATION('',(#1986),#3831);
#3869=PRODUCT_DEFINITION_CONTEXT('part definition',#3892,'design');
#3876=PRODUCT_DEFINITION('2026-10-07-08-56-00-255','Wheel_Holder',#3883,
#3869);
#3883=PRODUCT_DEFINITION_FORMATION('',$,#3900);
#3892=APPLICATION_CONTEXT(
'Core Data for Automotive Mechanical Design Process');
#3893=PRODUCT_CONTEXT('part definition',#3892,'mechanical');
#3900=PRODUCT('2026-10-07-08-56-00-255','Wheel_Holder',$,(#3893));
#3906=PRESENTATION_STYLE_ASSIGNMENT((#3912));
#3912=SURFACE_STYLE_USAGE(.BOTH.,#3918);
#3918=SURFACE_SIDE_STYLE('',(#3924));
#3924=SURFACE_STYLE_FILL_AREA(#3930);
#3930=FILL_AREA_STYLE('Opaque(248,135,1)',(#3936));
#3936=FILL_AREA_STYLE_COLOUR('Opaque(248,135,1)',#3942);
#3942=COLOUR_RGB('Opaque(248,135,1)', 0.08235294, 0.09019608, 0.10196078);
ENDSEC;
END-ISO-10303-21;
